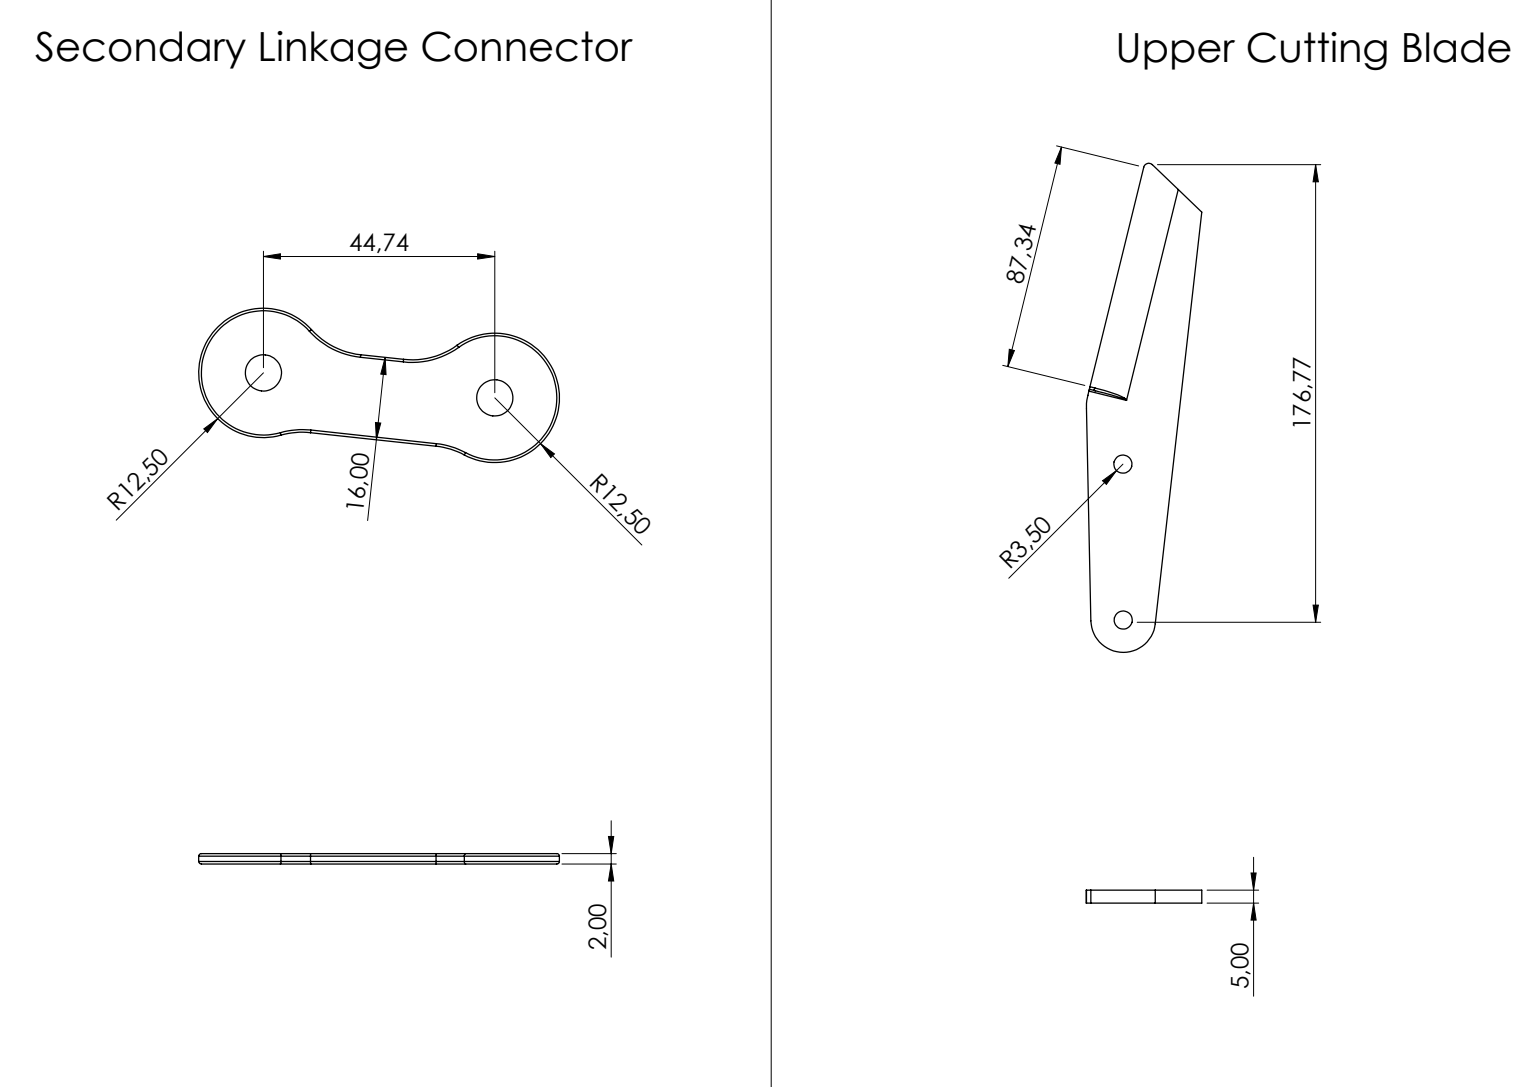
ISO-10303-21;
HEADER;
FILE_DESCRIPTION (('STEP AP214'),
    '1' );
FILE_NAME ('Secondary Linkage Connector.step',
    '2026-10-06T08:24:18',
    ( '' ),
    ( '' ),
    'SwSTEP 2.0',
    'SolidWorks 2020',
    '' );
FILE_SCHEMA (( 'AUTOMOTIVE_DESIGN' ));
ENDSEC;

DATA;
#3=AXIS2_PLACEMENT_3D ( 'NONE', #1835, #8382, #7525 ) ;
#18=CARTESIAN_POINT ( 'NONE',  ( -18.02719435607597021, -9.000000000000001776, -431.8467903975401896 ) ) ;
#24=VERTEX_POINT ( 'NONE', #8281 ) ;
#39=AXIS2_PLACEMENT_3D ( 'NONE', #1560, #10582, #8863 ) ;
#43=DIRECTION ( 'NONE',  ( 0.000000000000000000, -1.000000000000000000, 0.000000000000000000 ) ) ;
#51=CARTESIAN_POINT ( 'NONE',  ( -26.31853765676889267, -8.000000000000000000, -432.7407288192795249 ) ) ;
#69=CIRCLE ( 'NONE', #7777, 3.500000000000020428 ) ;
#75=ORIENTED_EDGE ( 'NONE', *, *, #5258, .T. ) ;
#94=EDGE_LOOP ( 'NONE', ( #5171, #2891 ) ) ;
#104=CARTESIAN_POINT ( 'NONE',  ( -46.74071243419621169, -8.000000000000000000, -414.3237589990241077 ) ) ;
#122=CARTESIAN_POINT ( 'NONE',  ( -46.74071243419621169, -8.000000000000000000, -414.3237589990241077 ) ) ;
#134=CYLINDRICAL_SURFACE ( 'NONE', #3984, 15.00000000000001776 ) ;
#162=ORIENTED_EDGE ( 'NONE', *, *, #3321, .F. ) ;
#168=VERTEX_POINT ( 'NONE', #2701 ) ;
#171=AXIS2_PLACEMENT_3D ( 'NONE', #4801, #2329, #8768 ) ;
#173=CYLINDRICAL_SURFACE ( 'NONE', #2650, 0.5000000000000004441 ) ;
#179=AXIS2_PLACEMENT_3D ( 'NONE', #8274, #10102, #4994 ) ;
#181=EDGE_CURVE ( 'NONE', #7240, #10131, #8649, .T. ) ;
#184=EDGE_CURVE ( 'NONE', #2293, #830, #6252, .T. ) ;
#204=CARTESIAN_POINT ( 'NONE',  ( -2.375181255485324439, -7.500000000000000888, -406.0201668106497550 ) ) ;
#222=DIRECTION ( 'NONE',  ( -0.9620620651437388204, 0.000000000000000000, 0.2728306852451987674 ) ) ;
#224=CARTESIAN_POINT ( 'NONE',  ( -48.08064548948741646, -8.000000000000000000, -401.8957833228595860 ) ) ;
#243=ORIENTED_EDGE ( 'NONE', *, *, #9605, .T. ) ;
#259=DIRECTION ( 'NONE',  ( -0.4716280258120416069, 0.000000000000000000, 0.8817975988108813779 ) ) ;
#262=AXIS2_PLACEMENT_3D ( 'NONE', #8998, #1740, #3461 ) ;
#280=DIRECTION ( 'NONE',  ( 0.000000000000000000, 1.000000000000000000, 0.000000000000000000 ) ) ;
#282=DIRECTION ( 'NONE',  ( 0.000000000000000000, 1.000000000000000000, 0.000000000000000000 ) ) ;
#295=PRODUCT_DEFINITION_SHAPE ( 'NONE', 'NONE',  #6660 ) ;
#318=ADVANCED_FACE ( 'NONE', ( #569 ), #2142, .T. ) ;
#322=ORIENTED_EDGE ( 'NONE', *, *, #2909, .F. ) ;
#329=ADVANCED_FACE ( 'NONE', ( #9439 ), #3687, .F. ) ;
#335=CIRCLE ( 'NONE', #1709, 15.00000000000001776 ) ;
#343=CARTESIAN_POINT ( 'NONE',  ( -43.33032886859687949, -9.000000000000001776, -402.2979831847329706 ) ) ;
#346=AXIS2_PLACEMENT_3D ( 'NONE', #860, #2744, #910 ) ;
#359=DIRECTION ( 'NONE',  ( 0.000000000000000000, 1.000000000000000000, 0.000000000000000000 ) ) ;
#372=CIRCLE ( 'NONE', #1744, 14.99999999999999467 ) ;
#384=LINE ( 'NONE', #2047, #7288 ) ;
#396=DIRECTION ( 'NONE',  ( -0.1071946444232961260, 0.000000000000000000, 0.9942380540931650135 ) ) ;
#398=ORIENTED_EDGE ( 'NONE', *, *, #3468, .T. ) ;
#410=FILL_AREA_STYLE_COLOUR ( '', #1992 ) ;
#421=STYLED_ITEM ( 'NONE', ( #698 ), #5138 ) ;
#451=CARTESIAN_POINT ( 'NONE',  ( -14.96977070983867009, -9.000000000000001776, -385.2505660326773409 ) ) ;
#460=ORIENTED_EDGE ( 'NONE', *, *, #1348, .F. ) ;
#463=DIRECTION ( 'NONE',  ( 0.000000000000000000, 1.000000000000000000, 0.000000000000000000 ) ) ;
#477=ADVANCED_FACE ( 'NONE', ( #9646 ), #582, .T. ) ;
#505=ADVANCED_FACE ( 'NONE', ( #3252 ), #1591, .F. ) ;
#511=VECTOR ( 'NONE', #4805, 1000.000000000000000 ) ;
#517=FACE_OUTER_BOUND ( 'NONE', #2695, .T. ) ;
#533=DIRECTION ( 'NONE',  ( 0.000000000000000000, -1.000000000000000000, 0.000000000000000000 ) ) ;
#543=EDGE_CURVE ( 'NONE', #1717, #2787, #7203, .T. ) ;
#554=EDGE_CURVE ( 'NONE', #2675, #1542, #4062, .T. ) ;
#565=ORIENTED_EDGE ( 'NONE', *, *, #5258, .F. ) ;
#569=FACE_OUTER_BOUND ( 'NONE', #2442, .T. ) ;
#570=CIRCLE ( 'NONE', #6572, 15.50000000000002487 ) ;
#582=TOROIDAL_SURFACE ( 'NONE', #1960, 12.00000000000000000, 0.5000000000000000000 ) ;
#597=EDGE_CURVE ( 'NONE', #10408, #168, #5818, .T. ) ;
#620=ORIENTED_EDGE ( 'NONE', *, *, #682, .T. ) ;
#622=ORIENTED_EDGE ( 'NONE', *, *, #10050, .T. ) ;
#641=EDGE_CURVE ( 'NONE', #5506, #9376, #3255, .T. ) ;
#647=ORIENTED_EDGE ( 'NONE', *, *, #4458, .T. ) ;
#652=CIRCLE ( 'NONE', #5110, 12.50000000000002309 ) ;
#661=VERTEX_POINT ( 'NONE', #3239 ) ;
#668=LINE ( 'NONE', #3943, #1019 ) ;
#671=ORIENTED_EDGE ( 'NONE', *, *, #1195, .T. ) ;
#682=EDGE_CURVE ( 'NONE', #9376, #10131, #2383, .T. ) ;
#685=ORIENTED_EDGE ( 'NONE', *, *, #8921, .F. ) ;
#692=AXIS2_PLACEMENT_3D ( 'NONE', #6618, #5963, #1017 ) ;
#697=FACE_OUTER_BOUND ( 'NONE', #8610, .T. ) ;
#698=PRESENTATION_STYLE_ASSIGNMENT (( #6324 ) ) ;
#739=EDGE_LOOP ( 'NONE', ( #961, #10607, #7941, #3569 ) ) ;
#764=ORIENTED_EDGE ( 'NONE', *, *, #7485, .F. ) ;
#767=AXIS2_PLACEMENT_3D ( 'NONE', #8861, #5631, #3922 ) ;
#775=AXIS2_PLACEMENT_3D ( 'NONE', #6193, #1570, #9735 ) ;
#780=EDGE_LOOP ( 'NONE', ( #4389, #3578, #5980, #685 ) ) ;
#784=STYLED_ITEM ( 'NONE', ( #5890 ), #966 ) ;
#801=DIRECTION ( 'NONE',  ( -0.9942380540931650135, 0.000000000000000000, -0.1071946444232960011 ) ) ;
#809=DIRECTION ( 'NONE',  ( 0.000000000000000000, 1.000000000000000000, 0.000000000000000000 ) ) ;
#814=DIRECTION ( 'NONE',  ( -0.4716280258120419955, 0.000000000000000000, 0.8817975988108811558 ) ) ;
#830=VERTEX_POINT ( 'NONE', #9310 ) ;
#832=DIRECTION ( 'NONE',  ( -0.5969176327498910695, 0.000000000000000000, -0.8023025238102309276 ) ) ;
#844=CARTESIAN_POINT ( 'NONE',  ( -27.92645732311833129, -8.000000000000000000, -417.8271580078820762 ) ) ;
#854=ORIENTED_EDGE ( 'NONE', *, *, #8756, .F. ) ;
#860=CARTESIAN_POINT ( 'NONE',  ( -37.82921798586427542, -8.000000000000000000, -422.3602549205905916 ) ) ;
#881=DIRECTION ( 'NONE',  ( 1.235123114895485641E-12, 1.000000000000000000, 4.329869796038106469E-12 ) ) ;
#882=DIRECTION ( 'NONE',  ( 0.000000000000000000, -1.000000000000000000, 0.000000000000000000 ) ) ;
#893=DIRECTION ( 'NONE',  ( 0.000000000000000000, 1.000000000000000000, 0.000000000000000000 ) ) ;
#899=EDGE_CURVE ( 'NONE', #830, #7069, #5948, .T. ) ;
#905=ORIENTED_EDGE ( 'NONE', *, *, #10218, .F. ) ;
#910=DIRECTION ( 'NONE',  ( 0.000000000000000000, 1.000000000000000000, 0.000000000000000000 ) ) ;
#911=VERTEX_POINT ( 'NONE', #2564 ) ;
#924=AXIS2_PLACEMENT_3D ( 'NONE', #8563, #5191, #9486 ) ;
#930=ORIENTED_EDGE ( 'NONE', *, *, #1348, .T. ) ;
#945=CARTESIAN_POINT ( 'NONE',  ( -2.000000000003786749, -9.500000000000001776, -409.4999999999758415 ) ) ;
#950=FACE_OUTER_BOUND ( 'NONE', #7230, .T. ) ;
#961=ORIENTED_EDGE ( 'NONE', *, *, #4838, .F. ) ;
#966=ADVANCED_BREP_SHAPE_REPRESENTATION ( '', ( #5138, #2817 ), #4734 ) ;
#1013=ADVANCED_FACE ( 'NONE', ( #6200 ), #2833, .T. ) ;
#1017=DIRECTION ( 'NONE',  ( 0.000000000000000000, 1.000000000000000000, 0.000000000000000000 ) ) ;
#1019=VECTOR ( 'NONE', #2386, 1000.000000000000000 ) ;
#1026=CARTESIAN_POINT ( 'NONE',  ( -9.285088343672491362, -8.000000000000000000, -419.6576319988688510 ) ) ;
#1033=VERTEX_POINT ( 'NONE', #10135 ) ;
#1038=CARTESIAN_POINT ( 'NONE',  ( -46.74071243419621169, -7.500000000000000888, -414.3237589990241077 ) ) ;
#1060=AXIS2_PLACEMENT_3D ( 'NONE', #4551, #2843, #6059 ) ;
#1077=CARTESIAN_POINT ( 'NONE',  ( -26.31853765676889267, -9.000000000000001776, -432.7407288192795249 ) ) ;
#1081=FACE_OUTER_BOUND ( 'NONE', #780, .T. ) ;
#1089=CARTESIAN_POINT ( 'NONE',  ( -2.000000000003786749, -9.500000000000001776, -409.4999999999758415 ) ) ;
#1096=EDGE_CURVE ( 'NONE', #4161, #1542, #7598, .T. ) ;
#1109=APPLICATION_CONTEXT ( 'automotive_design' ) ;
#1123=LINE ( 'NONE', #1174, #4934 ) ;
#1134=CARTESIAN_POINT ( 'NONE',  ( -27.98005464532998232, -9.000000000000001776, -417.3300389808354680 ) ) ;
#1146=EDGE_CURVE ( 'NONE', #2810, #4863, #5556, .T. ) ;
#1160=EDGE_CURVE ( 'NONE', #2578, #830, #10540, .T. ) ;
#1164=SHAPE_REPRESENTATION_RELATIONSHIP ( 'NONE' , 'NONE' ,  #1739, #966 ) ;
#1174=CARTESIAN_POINT ( 'NONE',  ( -48.08064548948741646, -9.500000000000001776, -401.8957833228595860 ) ) ;
#1183=VECTOR ( 'NONE', #6630, 1000.000000000000114 ) ;
#1195=EDGE_CURVE ( 'NONE', #661, #9639, #384, .T. ) ;
#1203=EDGE_CURVE ( 'NONE', #10408, #6648, #4023, .T. ) ;
#1243=AXIS2_PLACEMENT_3D ( 'NONE', #4932, #8161, #8048 ) ;
#1259=VERTEX_POINT ( 'NONE', #9314 ) ;
#1260=CARTESIAN_POINT ( 'NONE',  ( -13.30825372127758399, -7.500000000000000888, -400.6612558711213410 ) ) ;
#1265=CARTESIAN_POINT ( 'NONE',  ( -1.624818744522249503, -7.500000000000000888, -412.9798331893018712 ) ) ;
#1269=VECTOR ( 'NONE', #6090, 1000.000000000000114 ) ;
#1311=EDGE_LOOP ( 'NONE', ( #3567, #5407, #5270, #3199 ) ) ;
#1314=DIRECTION ( 'NONE',  ( 0.1071946444232958900, 0.000000000000000000, -0.9942380540931649024 ) ) ;
#1328=ADVANCED_FACE ( 'NONE', ( #5111 ), #6816, .T. ) ;
#1336=CYLINDRICAL_SURFACE ( 'NONE', #1965, 15.00000000000002309 ) ;
#1342=EDGE_LOOP ( 'NONE', ( #4527, #6060, #10354, #3368 ) ) ;
#1348=EDGE_CURVE ( 'NONE', #2010, #1489, #7829, .T. ) ;
#1356=AXIS2_PLACEMENT_3D ( 'NONE', #3266, #7300, #8854 ) ;
#1382=ORIENTED_EDGE ( 'NONE', *, *, #8963, .F. ) ;
#1392=AXIS2_PLACEMENT_3D ( 'NONE', #122, #8875, #3183 ) ;
#1403=CIRCLE ( 'NONE', #3292, 15.50000000000001421 ) ;
#1411=AXIS2_PLACEMENT_3D ( 'NONE', #1089, #7596, #5176 ) ;
#1426=EDGE_CURVE ( 'NONE', #10492, #1542, #5215, .T. ) ;
#1442=AXIS2_PLACEMENT_3D ( 'NONE', #2258, #3714, #7049 ) ;
#1449=AXIS2_PLACEMENT_3D ( 'NONE', #2696, #4307, #9306 ) ;
#1453=ORIENTED_EDGE ( 'NONE', *, *, #7309, .T. ) ;
#1462=DIRECTION ( 'NONE',  ( 0.000000000000000000, -1.000000000000000000, 0.000000000000000000 ) ) ;
#1486=CARTESIAN_POINT ( 'NONE',  ( -2.000000000003786749, -7.500000000000000888, -409.4999999999758415 ) ) ;
#1489=VERTEX_POINT ( 'NONE', #10527 ) ;
#1523=DIRECTION ( 'NONE',  ( 0.000000000000000000, 1.000000000000000000, 0.000000000000000000 ) ) ;
#1542=VERTEX_POINT ( 'NONE', #6029 ) ;
#1555=DIRECTION ( 'NONE',  ( 0.000000000000000000, 1.000000000000000000, 0.000000000000000000 ) ) ;
#1558=DIRECTION ( 'NONE',  ( 0.5828070674935411644, 0.000000000000000000, 0.8126105599114368250 ) ) ;
#1560=CARTESIAN_POINT ( 'NONE',  ( -2.000000000003786749, -7.500000000000000888, -409.4999999999758415 ) ) ;
#1570=DIRECTION ( 'NONE',  ( 0.000000000000000000, 1.000000000000000000, 0.000000000000000000 ) ) ;
#1581=CIRCLE ( 'NONE', #2784, 0.5000000000000004441 ) ;
#1591=CYLINDRICAL_SURFACE ( 'NONE', #6329, 3.500000000000020428 ) ;
#1611=FACE_BOUND ( 'NONE', #3102, .T. ) ;
#1613=( NAMED_UNIT ( * ) PLANE_ANGLE_UNIT ( ) SI_UNIT ( $, .RADIAN. ) );
#1624=CARTESIAN_POINT ( 'NONE',  ( -14.96977070983867009, -9.000000000000001776, -385.2505660326773409 ) ) ;
#1652=DIRECTION ( 'NONE',  ( -0.1071946444232959594, 0.000000000000000000, 0.9942380540931649024 ) ) ;
#1655=EDGE_LOOP ( 'NONE', ( #322, #8238, #1851, #243 ) ) ;
#1662=FACE_BOUND ( 'NONE', #3043, .T. ) ;
#1678=AXIS2_PLACEMENT_3D ( 'NONE', #9635, #3832, #396 ) ;
#1690=DIRECTION ( 'NONE',  ( 0.1071946444232947937, 0.000000000000000000, -0.9942380540931651245 ) ) ;
#1694=EDGE_CURVE ( 'NONE', #7772, #4372, #1906, .T. ) ;
#1709=AXIS2_PLACEMENT_3D ( 'NONE', #18, #1523, #3137 ) ;
#1710=VECTOR ( 'NONE', #4006, 1000.000000000000000 ) ;
#1717=VERTEX_POINT ( 'NONE', #3883 ) ;
#1739=SHAPE_REPRESENTATION ( 'Secondary Linkage Connector', ( #2817 ), #4734 ) ;
#1740=DIRECTION ( 'NONE',  ( 0.000000000000000000, 1.000000000000000000, 0.000000000000000000 ) ) ;
#1744=AXIS2_PLACEMENT_3D ( 'NONE', #451, #8713, #4585 ) ;
#1770=ORIENTED_EDGE ( 'NONE', *, *, #4366, .T. ) ;
#1782=AXIS2_PLACEMENT_3D ( 'NONE', #9436, #9485, #2981 ) ;
#1788=TOROIDAL_SURFACE ( 'NONE', #9510, 15.50000000000000000, 0.5000000000000000000 ) ;
#1795=AXIS2_PLACEMENT_3D ( 'NONE', #9777, #7308, #1558 ) ;
#1825=LINE ( 'NONE', #5841, #9195 ) ;
#1835=CARTESIAN_POINT ( 'NONE',  ( -37.82921798586427542, -9.000000000000001776, -422.3602549205905916 ) ) ;
#1851=ORIENTED_EDGE ( 'NONE', *, *, #10227, .T. ) ;
#1858=AXIS2_PLACEMENT_3D ( 'NONE', #7847, #8650, #4626 ) ;
#1861=ORIENTED_EDGE ( 'NONE', *, *, #7909, .T. ) ;
#1880=EDGE_CURVE ( 'NONE', #10437, #4923, #3628, .T. ) ;
#1888=VECTOR ( 'NONE', #9928, 1000.000000000000000 ) ;
#1904=DIRECTION ( 'NONE',  ( -0.5828070674935416084, 0.000000000000000000, -0.8126105599114364919 ) ) ;
#1906=CIRCLE ( 'NONE', #4643, 0.5000000000000004441 ) ;
#1921=ADVANCED_FACE ( 'NONE', ( #4094 ), #2768, .T. ) ;
#1942=DIRECTION ( 'NONE',  ( -0.8126105599114364919, 6.772514207610136972E-17, 0.5828070674935419415 ) ) ;
#1945=AXIS2_PLACEMENT_3D ( 'NONE', #7118, #3996, #10385 ) ;
#1960=AXIS2_PLACEMENT_3D ( 'NONE', #9757, #2288, #832 ) ;
#1965=AXIS2_PLACEMENT_3D ( 'NONE', #2797, #6170, #4507 ) ;
#1971=ORIENTED_EDGE ( 'NONE', *, *, #10530, .T. ) ;
#1975=CIRCLE ( 'NONE', #4723, 15.50000000000001421 ) ;
#1978=SURFACE_SIDE_STYLE ('',( #6922 ) ) ;
#1989=CARTESIAN_POINT ( 'NONE',  ( -1.624818744522249503, -7.500000000000000888, -412.9798331893018712 ) ) ;
#1990=CARTESIAN_POINT ( 'NONE',  ( -47.11589368967775471, -7.500000000000000888, -410.8439258096980780 ) ) ;
#1992=COLOUR_RGB ( '', 0.31764706, 0.68627451, 0.89019608) ;
#2010=VERTEX_POINT ( 'NONE', #4526 ) ;
#2013=EDGE_CURVE ( 'NONE', #9376, #2675, #372, .T. ) ;
#2022=CARTESIAN_POINT ( 'NONE',  ( -46.74071243419621169, -9.500000000000001776, -414.3237589990241077 ) ) ;
#2037=ADVANCED_FACE ( 'NONE', ( #2063 ), #7167, .T. ) ;
#2042=FACE_OUTER_BOUND ( 'NONE', #7532, .T. ) ;
#2047=CARTESIAN_POINT ( 'NONE',  ( -13.30825372127758399, -9.500000000000001776, -400.6612558711213410 ) ) ;
#2050=AXIS2_PLACEMENT_3D ( 'NONE', #9959, #2545, #7644 ) ;
#2058=ORIENTED_EDGE ( 'NONE', *, *, #6274, .F. ) ;
#2059=CARTESIAN_POINT ( 'NONE',  ( -37.62994892358009480, -8.000000000000000000, -402.7806230189665371 ) ) ;
#2063=FACE_OUTER_BOUND ( 'NONE', #3743, .T. ) ;
#2101=EDGE_LOOP ( 'NONE', ( #7660, #1453, #460, #3857 ) ) ;
#2121=CIRCLE ( 'NONE', #9340, 12.49999999999998934 ) ;
#2122=EDGE_LOOP ( 'NONE', ( #565, #7254, #9589, #2187 ) ) ;
#2123=CARTESIAN_POINT ( 'NONE',  ( -19.63511402242740189, -9.000000000000001776, -416.9332195861429113 ) ) ;
#2136=ORIENTED_EDGE ( 'NONE', *, *, #597, .T. ) ;
#2141=CIRCLE ( 'NONE', #1449, 12.49999999999998934 ) ;
#2142=TOROIDAL_SURFACE ( 'NONE', #4724, 15.50000000000000000, 0.5000000000000000000 ) ;
#2144=DIRECTION ( 'NONE',  ( 0.000000000000000000, 1.000000000000000000, 0.000000000000000000 ) ) ;
#2169=DIRECTION ( 'NONE',  ( 0.000000000000000000, 1.000000000000000000, 0.000000000000000000 ) ) ;
#2187=ORIENTED_EDGE ( 'NONE', *, *, #1880, .F. ) ;
#2199=CARTESIAN_POINT ( 'NONE',  ( -19.53582934753526246, -8.000000000000000000, -416.4196174530124495 ) ) ;
#2202=ADVANCED_FACE ( 'NONE', ( #8340 ), #10258, .T. ) ;
#2226=CIRCLE ( 'NONE', #2050, 0.5000000000000004441 ) ;
#2229=ORIENTED_EDGE ( 'NONE', *, *, #7954, .F. ) ;
#2244=AXIS2_PLACEMENT_3D ( 'NONE', #6985, #4554, #7828 ) ;
#2258=CARTESIAN_POINT ( 'NONE',  ( -13.30825372127758399, -8.000000000000000000, -400.6612558711213410 ) ) ;
#2280=DIRECTION ( 'NONE',  ( -0.1071946444232947937, 0.000000000000000000, 0.9942380540931651245 ) ) ;
#2288=DIRECTION ( 'NONE',  ( 0.000000000000000000, 1.000000000000000000, 0.000000000000000000 ) ) ;
#2293=VERTEX_POINT ( 'NONE', #8541 ) ;
#2296=ORIENTED_EDGE ( 'NONE', *, *, #6736, .F. ) ;
#2303=DIRECTION ( 'NONE',  ( 0.7508065140037780694, 0.000000000000000000, -0.6605222013903048195 ) ) ;
#2307=DIRECTION ( 'NONE',  ( 0.000000000000000000, -1.000000000000000000, 0.000000000000000000 ) ) ;
#2309=VECTOR ( 'NONE', #9307, 1000.000000000000114 ) ;
#2310=EDGE_LOOP ( 'NONE', ( #7345, #2928, #3923, #8777 ) ) ;
#2312=CIRCLE ( 'NONE', #8147, 15.00000000000001776 ) ;
#2327=ORIENTED_EDGE ( 'NONE', *, *, #5504, .F. ) ;
#2329=DIRECTION ( 'NONE',  ( 0.000000000000000000, -1.000000000000000000, 0.000000000000000000 ) ) ;
#2344=DIRECTION ( 'NONE',  ( 0.000000000000000000, -1.000000000000000000, 0.000000000000000000 ) ) ;
#2346=EDGE_CURVE ( 'NONE', #5580, #3896, #652, .T. ) ;
#2361=DIRECTION ( 'NONE',  ( 0.000000000000000000, 1.000000000000000000, 0.000000000000000000 ) ) ;
#2374=PRODUCT_CONTEXT ( 'NONE', #6331, 'mechanical' ) ;
#2376=DIRECTION ( 'NONE',  ( -1.908117741397742798E-11, 1.000000000000000000, -2.057253813257758150E-12 ) ) ;
#2383=LINE ( 'NONE', #7908, #3600 ) ;
#2386=DIRECTION ( 'NONE',  ( 0.000000000000000000, 1.000000000000000000, 0.000000000000000000 ) ) ;
#2401=EDGE_LOOP ( 'NONE', ( #2136, #9614, #2229, #5792 ) ) ;
#2404=ORIENTED_EDGE ( 'NONE', *, *, #1426, .T. ) ;
#2415=PLANE ( 'NONE',  #9955 ) ;
#2436=ORIENTED_EDGE ( 'NONE', *, *, #7339, .F. ) ;
#2439=VECTOR ( 'NONE', #3583, 1000.000000000000000 ) ;
#2442=EDGE_LOOP ( 'NONE', ( #8291, #3143, #9082, #10187 ) ) ;
#2451=EDGE_CURVE ( 'NONE', #24, #10408, #6657, .T. ) ;
#2466=CARTESIAN_POINT ( 'NONE',  ( -43.33032886859687949, -9.000000000000001776, -402.2979831847329706 ) ) ;
#2470=FACE_OUTER_BOUND ( 'NONE', #8150, .T. ) ;
#2481=CLOSED_SHELL ( 'NONE', ( #6399, #2037, #5406, #10272, #3571, #4819, #505, #7275, #10422, #2202, #8950, #8172, #9099, #1013, #6359, #4140, #329, #1921, #3048, #6808, #3575, #4250, #9302, #9900, #9238, #477, #8750, #10156, #1328, #7265, #318, #5097, #8841, #8169 ) ) ;
#2482=CARTESIAN_POINT ( 'NONE',  ( -19.68871134463705985, -7.500000000000000888, -416.4361005590961327 ) ) ;
#2486=EDGE_LOOP ( 'NONE', ( #8430, #75, #5442, #5537 ) ) ;
#2489=CIRCLE ( 'NONE', #3689, 12.50000000000001421 ) ;
#2501=ORIENTED_EDGE ( 'NONE', *, *, #3654, .F. ) ;
#2544=AXIS2_PLACEMENT_3D ( 'NONE', #6737, #6079, #4316 ) ;
#2545=DIRECTION ( 'NONE',  ( -0.9942380540931650135, 0.000000000000000000, -0.1071946444232960011 ) ) ;
#2563=DIRECTION ( 'NONE',  ( 0.000000000000000000, -1.000000000000000000, 0.000000000000000000 ) ) ;
#2564=CARTESIAN_POINT ( 'NONE',  ( -37.82921798586438911, -9.500000000000001776, -422.3602549205895684 ) ) ;
#2578=VERTEX_POINT ( 'NONE', #9303 ) ;
#2580=VECTOR ( 'NONE', #5428, 1000.000000000000000 ) ;
#2587=ORIENTED_EDGE ( 'NONE', *, *, #3654, .T. ) ;
#2606=FACE_OUTER_BOUND ( 'NONE', #2310, .T. ) ;
#2626=SURFACE_STYLE_USAGE ( .BOTH. , #1978 ) ;
#2641=ORIENTED_EDGE ( 'NONE', *, *, #10218, .T. ) ;
#2648=ORIENTED_EDGE ( 'NONE', *, *, #899, .T. ) ;
#2650=AXIS2_PLACEMENT_3D ( 'NONE', #2199, #3708, #8535 ) ;
#2662=MECHANICAL_DESIGN_GEOMETRIC_PRESENTATION_REPRESENTATION('',(#421),#4379);
#2675=VERTEX_POINT ( 'NONE', #9253 ) ;
#2683=EDGE_CURVE ( 'NONE', #5580, #4923, #1123, .T. ) ;
#2695=EDGE_LOOP ( 'NONE', ( #10232, #9170, #8030, #5805 ) ) ;
#2696=CARTESIAN_POINT ( 'NONE',  ( -2.000000000003786749, -8.000000000000000000, -409.4999999999758415 ) ) ;
#2697=AXIS2_PLACEMENT_3D ( 'NONE', #6841, #10009, #5264 ) ;
#2699=CARTESIAN_POINT ( 'NONE',  ( -3.339933055294988851, -9.000000000000001776, -397.0720243238112630 ) ) ;
#2701=CARTESIAN_POINT ( 'NONE',  ( -43.33032886862778099, -8.000000000000000000, -402.2979831847262631 ) ) ;
#2724=ORIENTED_EDGE ( 'NONE', *, *, #3777, .T. ) ;
#2726=DIRECTION ( 'NONE',  ( -0.1071946444232964035, 0.000000000000000000, 0.9942380540931649024 ) ) ;
#2740=CIRCLE ( 'NONE', #1356, 12.49999999999998934 ) ;
#2744=DIRECTION ( 'NONE',  ( -0.6697079934638360266, 0.000000000000000000, -0.7426245373610022016 ) ) ;
#2747=CARTESIAN_POINT ( 'NONE',  ( -37.57635160138833896, -7.500000000000000888, -403.2777420460153053 ) ) ;
#2768=TOROIDAL_SURFACE ( 'NONE', #8769, 15.50000000000000000, 0.5000000000000000000 ) ;
#2775=DIRECTION ( 'NONE',  ( 0.000000000000000000, -1.000000000000000000, 0.000000000000000000 ) ) ;
#2784=AXIS2_PLACEMENT_3D ( 'NONE', #8277, #1942, #4205 ) ;
#2787=VERTEX_POINT ( 'NONE', #8633 ) ;
#2789=ORIENTED_EDGE ( 'NONE', *, *, #899, .F. ) ;
#2794=DIRECTION ( 'NONE',  ( 0.2728306852451984343, 0.000000000000000000, 0.9620620651437388204 ) ) ;
#2797=CARTESIAN_POINT ( 'NONE',  ( -26.31853765676889267, -9.633703999999999823, -432.7407288192795249 ) ) ;
#2810=VERTEX_POINT ( 'NONE', #1989 ) ;
#2817=AXIS2_PLACEMENT_3D ( 'NONE', #8634, #3966, #3161 ) ;
#2823=CIRCLE ( 'NONE', #8826, 15.00000000000001776 ) ;
#2833=CYLINDRICAL_SURFACE ( 'NONE', #924, 12.49999999999998757 ) ;
#2842=ORIENTED_EDGE ( 'NONE', *, *, #5598, .F. ) ;
#2843=DIRECTION ( 'NONE',  ( 0.000000000000000000, 1.000000000000000000, 0.000000000000000000 ) ) ;
#2852=DIRECTION ( 'NONE',  ( 0.000000000000000000, -1.000000000000000000, 0.000000000000000000 ) ) ;
#2866=ORIENTED_EDGE ( 'NONE', *, *, #7339, .T. ) ;
#2881=DIRECTION ( 'NONE',  ( 0.1173809667161562209, 0.000000000000000000, -0.9930869592602555862 ) ) ;
#2891=ORIENTED_EDGE ( 'NONE', *, *, #543, .F. ) ;
#2893=CARTESIAN_POINT ( 'NONE',  ( -39.23786858994942151, -8.000000000000000000, -387.8670522075712483 ) ) ;
#2909=EDGE_CURVE ( 'NONE', #2810, #1259, #8675, .T. ) ;
#2910=DIRECTION ( 'NONE',  ( 0.1071946444232954182, 0.000000000000000000, -0.9942380540931651245 ) ) ;
#2923=AXIS2_PLACEMENT_3D ( 'NONE', #2893, #9207, #8737 ) ;
#2928=ORIENTED_EDGE ( 'NONE', *, *, #10338, .F. ) ;
#2981=DIRECTION ( 'NONE',  ( -0.1071946444232958900, 0.000000000000000000, 0.9942380540931649024 ) ) ;
#3026=CARTESIAN_POINT ( 'NONE',  ( -37.62994892359998289, -8.000000000000000000, -402.7806230189686971 ) ) ;
#3043=EDGE_LOOP ( 'NONE', ( #7539, #5201 ) ) ;
#3048=ADVANCED_FACE ( 'NONE', ( #1081 ), #6843, .T. ) ;
#3051=LINE ( 'NONE', #6219, #4361 ) ;
#3053=CARTESIAN_POINT ( 'NONE',  ( -46.74071243419621169, -8.000000000000000000, -414.3237589990241077 ) ) ;
#3056=SURFACE_SIDE_STYLE ('',( #10414 ) ) ;
#3073=ORIENTED_EDGE ( 'NONE', *, *, #597, .F. ) ;
#3077=VERTEX_POINT ( 'NONE', #8542 ) ;
#3081=CIRCLE ( 'NONE', #7887, 0.5000000000000004441 ) ;
#3102=EDGE_LOOP ( 'NONE', ( #6612, #162 ) ) ;
#3110=ORIENTED_EDGE ( 'NONE', *, *, #7485, .T. ) ;
#3125=EDGE_CURVE ( 'NONE', #6593, #7069, #10600, .T. ) ;
#3137=DIRECTION ( 'NONE',  ( -0.1071946444232958900, 0.000000000000000000, 0.9942380540931649024 ) ) ;
#3143=ORIENTED_EDGE ( 'NONE', *, *, #10338, .T. ) ;
#3152=ORIENTED_EDGE ( 'NONE', *, *, #682, .F. ) ;
#3154=CARTESIAN_POINT ( 'NONE',  ( -7.895350322666780940, -9.000000000000001776, -398.4775300148504016 ) ) ;
#3161=DIRECTION ( 'NONE',  ( 1.000000000000000000, 0.000000000000000000, 0.000000000000000000 ) ) ;
#3169=ORIENTED_EDGE ( 'NONE', *, *, #3440, .F. ) ;
#3183=DIRECTION ( 'NONE',  ( 0.7426245373610016465, 0.000000000000000000, -0.6697079934638365817 ) ) ;
#3194=VERTEX_POINT ( 'NONE', #8590 ) ;
#3199=ORIENTED_EDGE ( 'NONE', *, *, #6021, .F. ) ;
#3219=DIRECTION ( 'NONE',  ( 0.1071946444232959872, 0.000000000000000000, -0.9942380540931649024 ) ) ;
#3232=FACE_OUTER_BOUND ( 'NONE', #2101, .T. ) ;
#3239=CARTESIAN_POINT ( 'NONE',  ( -13.30825372127758399, -9.500000000000001776, -400.6612558711213410 ) ) ;
#3252=FACE_OUTER_BOUND ( 'NONE', #1655, .T. ) ;
#3253=CARTESIAN_POINT ( 'NONE',  ( -19.63511402242541237, -8.000000000000000000, -416.9332195861426840 ) ) ;
#3255=CIRCLE ( 'NONE', #171, 12.50000000000001421 ) ;
#3266=CARTESIAN_POINT ( 'NONE',  ( -2.000000000003786749, -8.000000000000000000, -409.4999999999758415 ) ) ;
#3290=ORIENTED_EDGE ( 'NONE', *, *, #5385, .T. ) ;
#3292=AXIS2_PLACEMENT_3D ( 'NONE', #9308, #9094, #4410 ) ;
#3312=DIRECTION ( 'NONE',  ( 0.000000000000000000, -1.000000000000000000, 0.000000000000000000 ) ) ;
#3313=AXIS2_PLACEMENT_3D ( 'NONE', #4697, #9693, #2280 ) ;
#3321=EDGE_CURVE ( 'NONE', #1259, #3194, #7259, .T. ) ;
#3327=ORIENTED_EDGE ( 'NONE', *, *, #8756, .T. ) ;
#3343=CARTESIAN_POINT ( 'NONE',  ( -46.74071243419621169, -9.500000000000001776, -414.3237589990241077 ) ) ;
#3368=ORIENTED_EDGE ( 'NONE', *, *, #10050, .F. ) ;
#3381=DIRECTION ( 'NONE',  ( 0.000000000000000000, -1.000000000000000000, 0.000000000000000000 ) ) ;
#3407=ORIENTED_EDGE ( 'NONE', *, *, #9625, .F. ) ;
#3417=CARTESIAN_POINT ( 'NONE',  ( -8.993684809926110191, -7.500000000000000888, -419.2513267189134467 ) ) ;
#3420=ORIENTED_EDGE ( 'NONE', *, *, #1146, .F. ) ;
#3426=AXIS2_PLACEMENT_3D ( 'NONE', #9072, #43, #9879 ) ;
#3431=CARTESIAN_POINT ( 'NONE',  ( -14.96977070983867009, -8.000000000000000000, -385.2505660326773409 ) ) ;
#3438=ORIENTED_EDGE ( 'NONE', *, *, #6940, .F. ) ;
#3440=EDGE_CURVE ( 'NONE', #6553, #5580, #10334, .T. ) ;
#3461=DIRECTION ( 'NONE',  ( -0.4824394482813016416, 0.000000000000000000, 0.8759293229148304993 ) ) ;
#3468=EDGE_CURVE ( 'NONE', #5957, #2787, #9355, .T. ) ;
#3483=CIRCLE ( 'NONE', #6565, 12.50000000000001421 ) ;
#3488=TOROIDAL_SURFACE ( 'NONE', #9326, 15.50000000000000000, 0.5000000000000000000 ) ;
#3508=CARTESIAN_POINT ( 'NONE',  ( -8.993684809926110191, -9.000000000000001776, -419.2513267189134467 ) ) ;
#3512=CARTESIAN_POINT ( 'NONE',  ( -46.74071243419621169, -9.000000000000001776, -414.3237589990241077 ) ) ;
#3517=ORIENTED_EDGE ( 'NONE', *, *, #6082, .F. ) ;
#3532=ORIENTED_EDGE ( 'NONE', *, *, #8111, .T. ) ;
#3534=DIRECTION ( 'NONE',  ( 0.000000000000000000, 1.000000000000000000, 0.000000000000000000 ) ) ;
#3536=EDGE_CURVE ( 'NONE', #6553, #168, #9721, .T. ) ;
#3541=DIRECTION ( 'NONE',  ( 0.7426245373610016465, 0.000000000000000000, -0.6697079934638365817 ) ) ;
#3564=AXIS2_PLACEMENT_3D ( 'NONE', #8918, #5528, #5635 ) ;
#3567=ORIENTED_EDGE ( 'NONE', *, *, #7921, .T. ) ;
#3569=ORIENTED_EDGE ( 'NONE', *, *, #1096, .F. ) ;
#3571=ADVANCED_FACE ( 'NONE', ( #4883 ), #6381, .F. ) ;
#3575=ADVANCED_FACE ( 'NONE', ( #8209 ), #8789, .T. ) ;
#3578=ORIENTED_EDGE ( 'NONE', *, *, #1096, .T. ) ;
#3583=DIRECTION ( 'NONE',  ( 9.254477013072932692E-13, 1.000000000000000000, 9.977795243863814969E-14 ) ) ;
#3599=TOROIDAL_SURFACE ( 'NONE', #6328, 12.00000000000000000, 0.5000000000000000000 ) ;
#3600=VECTOR ( 'NONE', #5647, 1000.000000000000000 ) ;
#3622=CARTESIAN_POINT ( 'NONE',  ( -2.000000000003786749, -9.500000000000001776, -409.4999999999758415 ) ) ;
#3628=CIRCLE ( 'NONE', #1392, 12.50000000000001243 ) ;
#3654=EDGE_CURVE ( 'NONE', #1489, #3077, #3483, .T. ) ;
#3666=ORIENTED_EDGE ( 'NONE', *, *, #5598, .T. ) ;
#3675=AXIS2_PLACEMENT_3D ( 'NONE', #1134, #7690, #10109 ) ;
#3677=CIRCLE ( 'NONE', #1795, 15.00000000000002487 ) ;
#3683=LINE ( 'NONE', #2123, #2439 ) ;
#3687=CYLINDRICAL_SURFACE ( 'NONE', #4890, 14.99999999999999467 ) ;
#3689=AXIS2_PLACEMENT_3D ( 'NONE', #9599, #3959, #7239 ) ;
#3703=FACE_BOUND ( 'NONE', #94, .T. ) ;
#3708=DIRECTION ( 'NONE',  ( -0.9942380540931650135, 0.000000000000000000, -0.1071946444232960011 ) ) ;
#3713=CARTESIAN_POINT ( 'NONE',  ( -7.659536309752155603, -8.000000000000000000, -398.9184288142485570 ) ) ;
#3714=DIRECTION ( 'NONE',  ( 0.9942380540931650135, 0.000000000000000000, 0.1071946444232960011 ) ) ;
#3723=ORIENTED_EDGE ( 'NONE', *, *, #3440, .T. ) ;
#3732=ORIENTED_EDGE ( 'NONE', *, *, #1203, .T. ) ;
#3741=CARTESIAN_POINT ( 'NONE',  ( -45.40077937890500692, -9.500000000000001776, -426.7517346751886862 ) ) ;
#3743=EDGE_LOOP ( 'NONE', ( #3841, #3110, #8398, #3152 ) ) ;
#3751=CARTESIAN_POINT ( 'NONE',  ( -46.74071243419621169, -9.500000000000001776, -414.3237589990241077 ) ) ;
#3761=AXIS2_PLACEMENT_3D ( 'NONE', #9004, #6690, #881 ) ;
#3766=LINE ( 'NONE', #5483, #7208 ) ;
#3777=EDGE_CURVE ( 'NONE', #4923, #168, #8279, .T. ) ;
#3779=CIRCLE ( 'NONE', #2244, 0.5000000000000004441 ) ;
#3832=DIRECTION ( 'NONE',  ( 0.000000000000000000, 1.000000000000000000, 0.000000000000000000 ) ) ;
#3841=ORIENTED_EDGE ( 'NONE', *, *, #641, .F. ) ;
#3857=ORIENTED_EDGE ( 'NONE', *, *, #5482, .F. ) ;
#3861=TOROIDAL_SURFACE ( 'NONE', #262, 12.00000000000000000, 0.5000000000000000000 ) ;
#3880=FACE_OUTER_BOUND ( 'NONE', #4914, .T. ) ;
#3883=CARTESIAN_POINT ( 'NONE',  ( -46.36553117871467578, -9.500000000000001776, -417.8035921883502510 ) ) ;
#3896=VERTEX_POINT ( 'NONE', #6923 ) ;
#3922=DIRECTION ( 'NONE',  ( -0.1071946444232959872, 0.000000000000000000, 0.9942380540931649024 ) ) ;
#3923=ORIENTED_EDGE ( 'NONE', *, *, #4838, .T. ) ;
#3932=CARTESIAN_POINT ( 'NONE',  ( -37.62994892356022092, -9.000000000000001776, -402.7806230189644339 ) ) ;
#3933=DIRECTION ( 'NONE',  ( -0.9942380540931649024, 0.000000000000000000, -0.1071946444232959872 ) ) ;
#3943=CARTESIAN_POINT ( 'NONE',  ( -0.6600669447125852018, -9.500000000000001776, -421.9279756761403632 ) ) ;
#3946=CIRCLE ( 'NONE', #7551, 11.99999999999998401 ) ;
#3959=DIRECTION ( 'NONE',  ( 0.000000000000000000, -1.000000000000000000, 0.000000000000000000 ) ) ;
#3966=DIRECTION ( 'NONE',  ( 0.000000000000000000, 0.000000000000000000, 1.000000000000000000 ) ) ;
#3984=AXIS2_PLACEMENT_3D ( 'NONE', #6746, #9965, #5867 ) ;
#3993=AXIS2_PLACEMENT_3D ( 'NONE', #6988, #6165, #2794 ) ;
#3996=DIRECTION ( 'NONE',  ( -0.1071946444232959872, 0.000000000000000000, 0.9942380540931649024 ) ) ;
#4006=DIRECTION ( 'NONE',  ( -4.096342363382135256E-11, 1.000000000000000000, -4.416507306988328157E-12 ) ) ;
#4015=ORIENTED_EDGE ( 'NONE', *, *, #3777, .F. ) ;
#4023=CIRCLE ( 'NONE', #2697, 15.49999999999999467 ) ;
#4025=CARTESIAN_POINT ( 'NONE',  ( -24.37035621709999944, -9.500000000000001776, -411.9118794995000030 ) ) ;
#4029=ORIENTED_EDGE ( 'NONE', *, *, #8616, .T. ) ;
#4032=ORIENTED_EDGE ( 'NONE', *, *, #2909, .T. ) ;
#4062=LINE ( 'NONE', #4816, #1710 ) ;
#4091=CARTESIAN_POINT ( 'NONE',  ( -46.74071243419621169, -7.500000000000000888, -414.3237589990241077 ) ) ;
#4092=DIRECTION ( 'NONE',  ( 0.4806425702415767498, 0.000000000000000000, -0.8769165978994644117 ) ) ;
#4094=FACE_OUTER_BOUND ( 'NONE', #7595, .T. ) ;
#4102=UNCERTAINTY_MEASURE_WITH_UNIT (LENGTH_MEASURE( 1.000000000000000082E-05 ), #6052, 'distance_accuracy_value', 'NONE');
#4111=AXIS2_PLACEMENT_3D ( 'NONE', #8207, #8043, #5729 ) ;
#4140=ADVANCED_FACE ( 'NONE', ( #8135 ), #5544, .T. ) ;
#4161=VERTEX_POINT ( 'NONE', #3026 ) ;
#4162=DIRECTION ( 'NONE',  ( 0.000000000000000000, -1.000000000000000000, 0.000000000000000000 ) ) ;
#4174=EDGE_CURVE ( 'NONE', #5957, #5389, #7940, .T. ) ;
#4175=DIRECTION ( 'NONE',  ( 0.000000000000000000, -1.000000000000000000, 0.000000000000000000 ) ) ;
#4179=CARTESIAN_POINT ( 'NONE',  ( -28.19723202891387359, -9.000000000000001776, -417.3534541501846888 ) ) ;
#4181=CYLINDRICAL_SURFACE ( 'NONE', #3426, 3.500000000000020428 ) ;
#4195=AXIS2_PLACEMENT_3D ( 'NONE', #8562, #6046, #1314 ) ;
#4205=DIRECTION ( 'NONE',  ( -1.318389841742372130E-13, 1.000000000000000000, -2.220446049250311061E-13 ) ) ;
#4229=CARTESIAN_POINT ( 'NONE',  ( -14.96977070983867009, -7.500000000000000888, -385.2505660326773409 ) ) ;
#4250=ADVANCED_FACE ( 'NONE', ( #8211 ), #3488, .T. ) ;
#4307=DIRECTION ( 'NONE',  ( 0.000000000000000000, 1.000000000000000000, 0.000000000000000000 ) ) ;
#4316=DIRECTION ( 'NONE',  ( 0.000000000000000000, 1.000000000000000000, 0.000000000000000000 ) ) ;
#4325=CARTESIAN_POINT ( 'NONE',  ( -27.98005464532998232, -7.500000000000000888, -417.3300389808354680 ) ) ;
#4327=DIRECTION ( 'NONE',  ( 0.1071946444232954182, 0.000000000000000000, -0.9942380540931651245 ) ) ;
#4336=AXIS2_PLACEMENT_3D ( 'NONE', #3622, #6030, #1904 ) ;
#4350=VERTEX_POINT ( 'NONE', #5198 ) ;
#4361=VECTOR ( 'NONE', #7943, 1000.000000000000000 ) ;
#4366=EDGE_CURVE ( 'NONE', #8504, #4350, #570, .T. ) ;
#4367=CIRCLE ( 'NONE', #10365, 12.50000000000001243 ) ;
#4372=VERTEX_POINT ( 'NONE', #8263 ) ;
#4378=AXIS2_PLACEMENT_3D ( 'NONE', #945, #3312, #5775 ) ;
#4379=( GEOMETRIC_REPRESENTATION_CONTEXT ( 3 ) GLOBAL_UNCERTAINTY_ASSIGNED_CONTEXT ( ( #5921 ) ) GLOBAL_UNIT_ASSIGNED_CONTEXT ( ( #9665, #1613, #6498 ) ) REPRESENTATION_CONTEXT ( 'NONE', 'WORKASPACE' ) );
#4389=ORIENTED_EDGE ( 'NONE', *, *, #7954, .T. ) ;
#4392=DIRECTION ( 'NONE',  ( -0.1071946444232947937, 0.000000000000000000, 0.9942380540931651245 ) ) ;
#4405=PRODUCT_DEFINITION_FORMATION_WITH_SPECIFIED_SOURCE ( 'ANY', '', #10331, .NOT_KNOWN. ) ;
#4410=DIRECTION ( 'NONE',  ( -0.1071946444232959594, 0.000000000000000000, 0.9942380540931649024 ) ) ;
#4417=PRODUCT_DEFINITION_CONTEXT ( 'detailed design', #1109, 'design' ) ;
#4419=ORIENTED_EDGE ( 'NONE', *, *, #181, .T. ) ;
#4439=CARTESIAN_POINT ( 'NONE',  ( -45.40077937890500692, -8.000000000000000000, -426.7517346751886862 ) ) ;
#4452=AXIS2_PLACEMENT_3D ( 'NONE', #9704, #2344, #5613 ) ;
#4455=DIRECTION ( 'NONE',  ( 0.2728306852451988784, 0.000000000000000000, 0.9620620651437385984 ) ) ;
#4458=EDGE_CURVE ( 'NONE', #1542, #10131, #2823, .T. ) ;
#4489=EDGE_CURVE ( 'NONE', #7069, #6915, #2312, .T. ) ;
#4507=DIRECTION ( 'NONE',  ( -0.7426245373610013134, 0.000000000000000000, 0.6697079934638370258 ) ) ;
#4510=DIRECTION ( 'NONE',  ( 0.8817975988108817109, 0.000000000000000000, 0.4716280258120411073 ) ) ;
#4526=CARTESIAN_POINT ( 'NONE',  ( -8.993684809926110191, -9.500000000000001776, -419.2513267189134467 ) ) ;
#4527=ORIENTED_EDGE ( 'NONE', *, *, #3125, .T. ) ;
#4542=VECTOR ( 'NONE', #6823, 1000.000000000000000 ) ;
#4551=CARTESIAN_POINT ( 'NONE',  ( -26.31853765676889267, -9.500000000000001776, -432.7407288192795249 ) ) ;
#4554=DIRECTION ( 'NONE',  ( -0.9942380540931650135, 0.000000000000000000, -0.1071946444232960011 ) ) ;
#4585=DIRECTION ( 'NONE',  ( 0.4716280258120412183, 0.000000000000000000, -0.8817975988108815999 ) ) ;
#4603=LINE ( 'NONE', #3741, #4542 ) ;
#4626=DIRECTION ( 'NONE',  ( 0.000000000000000000, 1.000000000000000000, 0.000000000000000000 ) ) ;
#4635=VERTEX_POINT ( 'NONE', #3253 ) ;
#4637=AXIS2_PLACEMENT_3D ( 'NONE', #7576, #7630, #5849 ) ;
#4643=AXIS2_PLACEMENT_3D ( 'NONE', #8656, #8764, #5485 ) ;
#4665=ORIENTED_EDGE ( 'NONE', *, *, #1694, .F. ) ;
#4666=CIRCLE ( 'NONE', #1060, 15.50000000000000711 ) ;
#4679=DIRECTION ( 'NONE',  ( 0.000000000000000000, -1.000000000000000000, 0.000000000000000000 ) ) ;
#4697=CARTESIAN_POINT ( 'NONE',  ( -46.74071243419621169, -7.500000000000000888, -414.3237589990241077 ) ) ;
#4700=VECTOR ( 'NONE', #2563, 1000.000000000000000 ) ;
#4701=ORIENTED_EDGE ( 'NONE', *, *, #7615, .T. ) ;
#4723=AXIS2_PLACEMENT_3D ( 'NONE', #5674, #5624, #1652 ) ;
#4724=AXIS2_PLACEMENT_3D ( 'NONE', #5292, #359, #2881 ) ;
#4725=ORIENTED_EDGE ( 'NONE', *, *, #2683, .F. ) ;
#4731=PLANE ( 'NONE',  #767 ) ;
#4734=( GEOMETRIC_REPRESENTATION_CONTEXT ( 3 ) GLOBAL_UNCERTAINTY_ASSIGNED_CONTEXT ( ( #5168 ) ) GLOBAL_UNIT_ASSIGNED_CONTEXT ( ( #9021, #9074, #9772 ) ) REPRESENTATION_CONTEXT ( 'NONE', 'WORKASPACE' ) );
#4741=SHAPE_DEFINITION_REPRESENTATION ( #295, #1739 ) ;
#4743=DIRECTION ( 'NONE',  ( 0.1071946444232947937, 0.000000000000000000, -0.9942380540931651245 ) ) ;
#4744=DIRECTION ( 'NONE',  ( 0.000000000000000000, 1.000000000000000000, 0.000000000000000000 ) ) ;
#4763=DIRECTION ( 'NONE',  ( 0.1071946444232954182, 0.000000000000000000, -0.9942380540931651245 ) ) ;
#4770=ORIENTED_EDGE ( 'NONE', *, *, #9491, .F. ) ;
#4785=FACE_OUTER_BOUND ( 'NONE', #9875, .T. ) ;
#4801=CARTESIAN_POINT ( 'NONE',  ( -2.000000000003786749, -9.000000000000001776, -409.4999999999758415 ) ) ;
#4805=DIRECTION ( 'NONE',  ( 0.000000000000000000, 1.000000000000000000, 0.000000000000000000 ) ) ;
#4809=CIRCLE ( 'NONE', #3, 0.5000000000000004441 ) ;
#4816=CARTESIAN_POINT ( 'NONE',  ( -13.36185104352900055, -9.000000000000001776, -400.1641368440791098 ) ) ;
#4818=CIRCLE ( 'NONE', #7874, 11.99999999999997691 ) ;
#4819=ADVANCED_FACE ( 'NONE', ( #3880 ), #9624, .F. ) ;
#4832=DIRECTION ( 'NONE',  ( 0.000000000000000000, 1.000000000000000000, 0.000000000000000000 ) ) ;
#4838=EDGE_CURVE ( 'NONE', #10018, #4161, #7368, .T. ) ;
#4850=VECTOR ( 'NONE', #10464, 1000.000000000000000 ) ;
#4861=ORIENTED_EDGE ( 'NONE', *, *, #5217, .T. ) ;
#4863=VERTEX_POINT ( 'NONE', #6508 ) ;
#4867=DIRECTION ( 'NONE',  ( 0.000000000000000000, -1.000000000000000000, 0.000000000000000000 ) ) ;
#4880=CIRCLE ( 'NONE', #5730, 0.5000000000000004441 ) ;
#4883=FACE_OUTER_BOUND ( 'NONE', #7809, .T. ) ;
#4889=AXIS2_PLACEMENT_3D ( 'NONE', #10415, #7253, #8972 ) ;
#4890=AXIS2_PLACEMENT_3D ( 'NONE', #6152, #463, #7078 ) ;
#4897=CYLINDRICAL_SURFACE ( 'NONE', #7415, 12.49999999999998757 ) ;
#4906=EDGE_CURVE ( 'NONE', #7180, #6903, #2141, .T. ) ;
#4914=EDGE_LOOP ( 'NONE', ( #10318, #2058, #9814, #9399 ) ) ;
#4923=VERTEX_POINT ( 'NONE', #224 ) ;
#4932=CARTESIAN_POINT ( 'NONE',  ( -46.74071243419621169, -7.500000000000000888, -414.3237589990241077 ) ) ;
#4934=VECTOR ( 'NONE', #2144, 1000.000000000000000 ) ;
#4976=ORIENTED_EDGE ( 'NONE', *, *, #1146, .T. ) ;
#4994=DIRECTION ( 'NONE',  ( -6.262351748276267552E-13, -1.000000000000000000, 1.110223024625155531E-12 ) ) ;
#5035=DIRECTION ( 'NONE',  ( -0.5828070674935414974, 0.000000000000000000, -0.8126105599114366029 ) ) ;
#5048=COLOUR_RGB ( '', 0.31764706, 0.68627451, 0.89019608) ;
#5058=AXIS2_PLACEMENT_3D ( 'NONE', #4229, #4175, #7449 ) ;
#5083=DIRECTION ( 'NONE',  ( 0.2896000924642900820, 0.000000000000000000, 0.9571477349106952692 ) ) ;
#5097=ADVANCED_FACE ( 'NONE', ( #2042 ), #8582, .T. ) ;
#5102=CARTESIAN_POINT ( 'NONE',  ( -43.46674421124934184, -9.000000000000001776, -402.7790142173016648 ) ) ;
#5110=AXIS2_PLACEMENT_3D ( 'NONE', #6999, #10271, #5366 ) ;
#5111=FACE_OUTER_BOUND ( 'NONE', #1311, .T. ) ;
#5136=CARTESIAN_POINT ( 'NONE',  ( -27.92645732311634532, -9.000000000000001776, -417.8271580078818488 ) ) ;
#5138=MANIFOLD_SOLID_BREP ( 'Stock-MAS-686-1', #2481 ) ;
#5168=UNCERTAINTY_MEASURE_WITH_UNIT (LENGTH_MEASURE( 1.000000000000000082E-05 ), #9021, 'distance_accuracy_value', 'NONE');
#5169=DIRECTION ( 'NONE',  ( 0.000000000000000000, -1.000000000000000000, 0.000000000000000000 ) ) ;
#5171=ORIENTED_EDGE ( 'NONE', *, *, #10479, .F. ) ;
#5176=DIRECTION ( 'NONE',  ( -0.1071946444232961260, 0.000000000000000000, 0.9942380540931650135 ) ) ;
#5181=VECTOR ( 'NONE', #9561, 1000.000000000000114 ) ;
#5185=ORIENTED_EDGE ( 'NONE', *, *, #641, .T. ) ;
#5191=DIRECTION ( 'NONE',  ( 0.000000000000000000, 1.000000000000000000, 0.000000000000000000 ) ) ;
#5198=CARTESIAN_POINT ( 'NONE',  ( -19.68871134463705985, -7.500000000000000888, -416.4361005590961327 ) ) ;
#5201=ORIENTED_EDGE ( 'NONE', *, *, #6274, .T. ) ;
#5215=CIRCLE ( 'NONE', #1442, 0.5000000000000004441 ) ;
#5217=EDGE_CURVE ( 'NONE', #2675, #10018, #1825, .T. ) ;
#5258=EDGE_CURVE ( 'NONE', #3896, #10437, #4603, .T. ) ;
#5264=DIRECTION ( 'NONE',  ( -0.2728306852452879183, 0.000000000000000000, -0.9620620651437133963 ) ) ;
#5270=ORIENTED_EDGE ( 'NONE', *, *, #1160, .F. ) ;
#5274=CARTESIAN_POINT ( 'NONE',  ( -37.57635160138833896, -7.500000000000000888, -403.2777420460153053 ) ) ;
#5292=CARTESIAN_POINT ( 'NONE',  ( -39.23786858994942151, -9.000000000000001776, -387.8670522075712483 ) ) ;
#5294=( NAMED_UNIT ( * ) SI_UNIT ( $, .STERADIAN. ) SOLID_ANGLE_UNIT ( ) );
#5304=CIRCLE ( 'NONE', #8915, 12.50000000000002309 ) ;
#5349=AXIS2_PLACEMENT_3D ( 'NONE', #3053, #2361, #2303 ) ;
#5363=DIRECTION ( 'NONE',  ( 0.000000000000000000, 1.000000000000000000, 0.000000000000000000 ) ) ;
#5366=DIRECTION ( 'NONE',  ( 0.2728306852451984343, 0.000000000000000000, 0.9620620651437388204 ) ) ;
#5385=EDGE_CURVE ( 'NONE', #6619, #661, #5396, .T. ) ;
#5389=VERTEX_POINT ( 'NONE', #8926 ) ;
#5396=CIRCLE ( 'NONE', #775, 15.50000000000000711 ) ;
#5405=CARTESIAN_POINT ( 'NONE',  ( -37.45790571718422513, -8.000000000000000000, -422.6951089173222726 ) ) ;
#5406=ADVANCED_FACE ( 'NONE', ( #10591 ), #4897, .T. ) ;
#5407=ORIENTED_EDGE ( 'NONE', *, *, #184, .T. ) ;
#5428=DIRECTION ( 'NONE',  ( 1.881029090955282852E-11, 1.000000000000000000, 2.085935400224071097E-11 ) ) ;
#5442=ORIENTED_EDGE ( 'NONE', *, *, #9093, .F. ) ;
#5444=ORIENTED_EDGE ( 'NONE', *, *, #9625, .T. ) ;
#5456=ORIENTED_EDGE ( 'NONE', *, *, #10227, .F. ) ;
#5482=EDGE_CURVE ( 'NONE', #7772, #2010, #1403, .T. ) ;
#5483=CARTESIAN_POINT ( 'NONE',  ( -27.92645732311634532, -9.000000000000001776, -417.8271580078818488 ) ) ;
#5485=DIRECTION ( 'NONE',  ( 0.000000000000000000, -1.000000000000000000, 0.000000000000000000 ) ) ;
#5504=EDGE_CURVE ( 'NONE', #8504, #6903, #1581, .T. ) ;
#5506=VERTEX_POINT ( 'NONE', #2699 ) ;
#5520=CYLINDRICAL_SURFACE ( 'NONE', #4889, 12.49999999999998579 ) ;
#5528=DIRECTION ( 'NONE',  ( 0.000000000000000000, 1.000000000000000000, 0.000000000000000000 ) ) ;
#5537=ORIENTED_EDGE ( 'NONE', *, *, #8619, .F. ) ;
#5544=PLANE ( 'NONE',  #1945 ) ;
#5550=EDGE_LOOP ( 'NONE', ( #6256, #4029, #4665, #2842 ) ) ;
#5556=CIRCLE ( 'NONE', #8645, 3.500000000000020428 ) ;
#5580=VERTEX_POINT ( 'NONE', #10366 ) ;
#5598=EDGE_CURVE ( 'NONE', #2578, #7772, #6939, .T. ) ;
#5613=DIRECTION ( 'NONE',  ( 0.1071946444232947937, 0.000000000000000000, -0.9942380540931651245 ) ) ;
#5624=DIRECTION ( 'NONE',  ( 0.000000000000000000, -1.000000000000000000, 0.000000000000000000 ) ) ;
#5631=DIRECTION ( 'NONE',  ( 0.000000000000000000, 1.000000000000000000, 0.000000000000000000 ) ) ;
#5635=DIRECTION ( 'NONE',  ( 0.7426245373610527167, 0.000000000000000000, -0.6697079934637800713 ) ) ;
#5647=DIRECTION ( 'NONE',  ( -4.963222276338128250E-12, 1.000000000000000000, -2.652296088385032042E-12 ) ) ;
#5674=CARTESIAN_POINT ( 'NONE',  ( -26.31853765676889267, -7.500000000000000888, -432.7407288192795249 ) ) ;
#5701=VECTOR ( 'NONE', #533, 1000.000000000000000 ) ;
#5712=ORIENTED_EDGE ( 'NONE', *, *, #4458, .F. ) ;
#5729=DIRECTION ( 'NONE',  ( 0.1071946444232959594, 0.000000000000000000, -0.9942380540931649024 ) ) ;
#5730=AXIS2_PLACEMENT_3D ( 'NONE', #5912, #7634, #5852 ) ;
#5751=DIRECTION ( 'NONE',  ( -0.1071946444232964035, 0.000000000000000000, 0.9942380540931649024 ) ) ;
#5775=DIRECTION ( 'NONE',  ( -0.1071946444232954182, 0.000000000000000000, 0.9942380540931651245 ) ) ;
#5783=CARTESIAN_POINT ( 'NONE',  ( -2.000000000003786749, -9.000000000000001776, -409.4999999999758415 ) ) ;
#5786=DIRECTION ( 'NONE',  ( 0.000000000000000000, 1.000000000000000000, 0.000000000000000000 ) ) ;
#5792=ORIENTED_EDGE ( 'NONE', *, *, #1203, .F. ) ;
#5800=EDGE_CURVE ( 'NONE', #4863, #2810, #7923, .T. ) ;
#5805=ORIENTED_EDGE ( 'NONE', *, *, #9172, .F. ) ;
#5818=CIRCLE ( 'NONE', #3761, 0.5000000000000004441 ) ;
#5831=CARTESIAN_POINT ( 'NONE',  ( -3.339933055294988851, -8.000000000000000000, -397.0720243238112630 ) ) ;
#5840=DIRECTION ( 'NONE',  ( 0.5828070674935411644, 0.000000000000000000, 0.8126105599114369360 ) ) ;
#5841=CARTESIAN_POINT ( 'NONE',  ( -13.36185104352900055, -9.000000000000001776, -400.1641368440791098 ) ) ;
#5849=DIRECTION ( 'NONE',  ( -0.2728306852451987119, 0.000000000000000000, -0.9620620651437387094 ) ) ;
#5852=DIRECTION ( 'NONE',  ( 0.000000000000000000, -1.000000000000000000, 0.000000000000000000 ) ) ;
#5862=CARTESIAN_POINT ( 'NONE',  ( -19.68871134463705985, -9.500000000000001776, -416.4361005590961327 ) ) ;
#5867=DIRECTION ( 'NONE',  ( 0.1071946444232958900, 0.000000000000000000, -0.9942380540931649024 ) ) ;
#5890=PRESENTATION_STYLE_ASSIGNMENT (( #2626 ) ) ;
#5893=DIRECTION ( 'NONE',  ( 0.000000000000000000, -1.000000000000000000, 0.000000000000000000 ) ) ;
#5899=ORIENTED_EDGE ( 'NONE', *, *, #8111, .F. ) ;
#5912=CARTESIAN_POINT ( 'NONE',  ( -37.57635160138833896, -9.000000000000001776, -403.2777420460153053 ) ) ;
#5921=UNCERTAINTY_MEASURE_WITH_UNIT (LENGTH_MEASURE( 1.000000000000000082E-05 ), #9665, 'distance_accuracy_value', 'NONE');
#5931=( GEOMETRIC_REPRESENTATION_CONTEXT ( 3 ) GLOBAL_UNCERTAINTY_ASSIGNED_CONTEXT ( ( #4102 ) ) GLOBAL_UNIT_ASSIGNED_CONTEXT ( ( #6052, #9240, #5294 ) ) REPRESENTATION_CONTEXT ( 'NONE', 'WORKASPACE' ) );
#5947=CARTESIAN_POINT ( 'NONE',  ( -46.74071243419621169, -9.500000000000001776, -414.3237589990241077 ) ) ;
#5948=LINE ( 'NONE', #5136, #1888 ) ;
#5957=VERTEX_POINT ( 'NONE', #9300 ) ;
#5963=DIRECTION ( 'NONE',  ( 0.9942380540931650135, 0.000000000000000000, 0.1071946444232960011 ) ) ;
#5974=LINE ( 'NONE', #8285, #1183 ) ;
#5980=ORIENTED_EDGE ( 'NONE', *, *, #1426, .F. ) ;
#5985=LINE ( 'NONE', #8762, #2580 ) ;
#5994=FACE_OUTER_BOUND ( 'NONE', #5550, .T. ) ;
#6020=DIRECTION ( 'NONE',  ( -0.7494507079133034821, 0.000000000000000000, 0.6620601456123518247 ) ) ;
#6021=EDGE_CURVE ( 'NONE', #911, #2578, #4666, .T. ) ;
#6029=CARTESIAN_POINT ( 'NONE',  ( -13.36185104356876785, -8.000000000000000000, -400.1641368440833730 ) ) ;
#6030=DIRECTION ( 'NONE',  ( 0.000000000000000000, -1.000000000000000000, 0.000000000000000000 ) ) ;
#6046=DIRECTION ( 'NONE',  ( 0.000000000000000000, 1.000000000000000000, 0.000000000000000000 ) ) ;
#6052=( LENGTH_UNIT ( ) NAMED_UNIT ( * ) SI_UNIT ( .MILLI., .METRE. ) );
#6058=EDGE_LOOP ( 'NONE', ( #4770, #2866, #905, #764 ) ) ;
#6059=DIRECTION ( 'NONE',  ( -0.7426245373609573486, 0.000000000000000000, 0.6697079934638857646 ) ) ;
#6060=ORIENTED_EDGE ( 'NONE', *, *, #4489, .T. ) ;
#6069=LINE ( 'NONE', #10216, #6775 ) ;
#6079=DIRECTION ( 'NONE',  ( 0.9942380540931650135, 0.000000000000000000, 0.1071946444232960011 ) ) ;
#6082=EDGE_CURVE ( 'NONE', #4372, #4635, #3683, .T. ) ;
#6090=DIRECTION ( 'NONE',  ( 0.9942380540931649024, 0.000000000000000000, 0.1071946444232959872 ) ) ;
#6136=CYLINDRICAL_SURFACE ( 'NONE', #1411, 12.49999999999998579 ) ;
#6143=ORIENTED_EDGE ( 'NONE', *, *, #4174, .F. ) ;
#6152=CARTESIAN_POINT ( 'NONE',  ( -14.96977070983867009, -9.633703999999999823, -385.2505660326773409 ) ) ;
#6165=DIRECTION ( 'NONE',  ( 0.000000000000000000, -1.000000000000000000, 0.000000000000000000 ) ) ;
#6167=CIRCLE ( 'NONE', #692, 0.5000000000000004441 ) ;
#6170=DIRECTION ( 'NONE',  ( 0.000000000000000000, 1.000000000000000000, 0.000000000000000000 ) ) ;
#6179=CARTESIAN_POINT ( 'NONE',  ( -2.000000000003786749, -9.500000000000001776, -409.4999999999758415 ) ) ;
#6192=ORIENTED_EDGE ( 'NONE', *, *, #7629, .F. ) ;
#6193=CARTESIAN_POINT ( 'NONE',  ( -14.96977070983867009, -9.500000000000001776, -385.2505660326773409 ) ) ;
#6200=FACE_OUTER_BOUND ( 'NONE', #6607, .T. ) ;
#6208=AXIS2_PLACEMENT_3D ( 'NONE', #1038, #4162, #1690 ) ;
#6214=ORIENTED_EDGE ( 'NONE', *, *, #7921, .F. ) ;
#6219=CARTESIAN_POINT ( 'NONE',  ( -9.285088343770869557, -9.000000000000001776, -419.6576319987959778 ) ) ;
#6252=CIRCLE ( 'NONE', #9009, 15.00000000000002309 ) ;
#6256=ORIENTED_EDGE ( 'NONE', *, *, #1160, .T. ) ;
#6274=EDGE_CURVE ( 'NONE', #5389, #5957, #7424, .T. ) ;
#6299=AXIS2_PLACEMENT_3D ( 'NONE', #10010, #282, #8439 ) ;
#6324=SURFACE_STYLE_USAGE ( .BOTH. , #3056 ) ;
#6328=AXIS2_PLACEMENT_3D ( 'NONE', #6652, #6597, #5083 ) ;
#6329=AXIS2_PLACEMENT_3D ( 'NONE', #1486, #4867, #4763 ) ;
#6331=APPLICATION_CONTEXT ( 'automotive_design' ) ;
#6359=ADVANCED_FACE ( 'NONE', ( #2606 ), #134, .F. ) ;
#6381=CYLINDRICAL_SURFACE ( 'NONE', #1243, 3.500000000000020428 ) ;
#6399=ADVANCED_FACE ( 'NONE', ( #8503 ), #6136, .T. ) ;
#6412=ORIENTED_EDGE ( 'NONE', *, *, #8864, .F. ) ;
#6421=CARTESIAN_POINT ( 'NONE',  ( -26.31853765676889267, -8.000000000000000000, -432.7407288192795249 ) ) ;
#6458=ORIENTED_EDGE ( 'NONE', *, *, #6021, .T. ) ;
#6496=DIRECTION ( 'NONE',  ( -0.1071946444232959872, 0.000000000000000000, 0.9942380540931649024 ) ) ;
#6498=( NAMED_UNIT ( * ) SI_UNIT ( $, .STERADIAN. ) SOLID_ANGLE_UNIT ( ) );
#6502=ORIENTED_EDGE ( 'NONE', *, *, #3536, .T. ) ;
#6508=CARTESIAN_POINT ( 'NONE',  ( -2.375181255485324439, -7.500000000000000888, -406.0201668106497550 ) ) ;
#6522=ORIENTED_EDGE ( 'NONE', *, *, #4366, .F. ) ;
#6553=VERTEX_POINT ( 'NONE', #343 ) ;
#6562=CIRCLE ( 'NONE', #4336, 12.00000000000001243 ) ;
#6565=AXIS2_PLACEMENT_3D ( 'NONE', #5783, #3381, #5035 ) ;
#6567=EDGE_LOOP ( 'NONE', ( #9804, #4976 ) ) ;
#6572=AXIS2_PLACEMENT_3D ( 'NONE', #7514, #8320, #5840 ) ;
#6585=EDGE_CURVE ( 'NONE', #2010, #6619, #6562, .T. ) ;
#6593=VERTEX_POINT ( 'NONE', #4325 ) ;
#6597=DIRECTION ( 'NONE',  ( 0.000000000000000000, 1.000000000000000000, 0.000000000000000000 ) ) ;
#6607=EDGE_LOOP ( 'NONE', ( #4725, #3169, #6502, #4015 ) ) ;
#6610=AXIS2_PLACEMENT_3D ( 'NONE', #4091, #1462, #4743 ) ;
#6612=ORIENTED_EDGE ( 'NONE', *, *, #9605, .F. ) ;
#6618=CARTESIAN_POINT ( 'NONE',  ( -37.57635160138833896, -8.000000000000000000, -403.2777420460153053 ) ) ;
#6619=VERTEX_POINT ( 'NONE', #10170 ) ;
#6630=DIRECTION ( 'NONE',  ( -0.9942380540931649024, 0.000000000000000000, -0.1071946444232959872 ) ) ;
#6648=VERTEX_POINT ( 'NONE', #5274 ) ;
#6652=CARTESIAN_POINT ( 'NONE',  ( -46.74071243419621169, -9.000000000000001776, -414.3237589990241077 ) ) ;
#6657=CIRCLE ( 'NONE', #3564, 11.99999999999999289 ) ;
#6660=PRODUCT_DEFINITION ( 'UNKNOWN', '', #4405, #4417 ) ;
#6690=DIRECTION ( 'NONE',  ( 0.9620620651437388204, -2.527616691482515415E-15, -0.2728306852451987674 ) ) ;
#6710=DIRECTION ( 'NONE',  ( 0.1071946444232958900, 0.000000000000000000, -0.9942380540931649024 ) ) ;
#6730=DIRECTION ( 'NONE',  ( 0.000000000000000000, 1.000000000000000000, 0.000000000000000000 ) ) ;
#6736=EDGE_CURVE ( 'NONE', #7240, #8504, #4818, .T. ) ;
#6737=CARTESIAN_POINT ( 'NONE',  ( -37.72923359849013281, -8.000000000000000000, -403.2942251520989316 ) ) ;
#6742=ORIENTED_EDGE ( 'NONE', *, *, #9491, .T. ) ;
#6746=CARTESIAN_POINT ( 'NONE',  ( -39.23786858994942151, -9.633703999999999823, -387.8670522075712483 ) ) ;
#6761=FACE_OUTER_BOUND ( 'NONE', #2122, .T. ) ;
#6775=VECTOR ( 'NONE', #2852, 1000.000000000000000 ) ;
#6789=DIRECTION ( 'NONE',  ( -0.7426245373610013134, 0.000000000000000000, 0.6697079934638370258 ) ) ;
#6794=DIRECTION ( 'NONE',  ( 0.2728306852451984343, 0.000000000000000000, 0.9620620651437388204 ) ) ;
#6806=ORIENTED_EDGE ( 'NONE', *, *, #6585, .T. ) ;
#6808=ADVANCED_FACE ( 'NONE', ( #7092 ), #7562, .T. ) ;
#6816=TOROIDAL_SURFACE ( 'NONE', #8183, 15.50000000000000000, 0.5000000000000000000 ) ;
#6823=DIRECTION ( 'NONE',  ( 0.000000000000000000, 1.000000000000000000, 0.000000000000000000 ) ) ;
#6841=CARTESIAN_POINT ( 'NONE',  ( -39.23786858994942151, -7.500000000000000888, -387.8670522075712483 ) ) ;
#6843=CYLINDRICAL_SURFACE ( 'NONE', #2544, 0.5000000000000004441 ) ;
#6848=ORIENTED_EDGE ( 'NONE', *, *, #7668, .F. ) ;
#6871=FILL_AREA_STYLE ('',( #410 ) ) ;
#6877=ORIENTED_EDGE ( 'NONE', *, *, #6967, .T. ) ;
#6881=CIRCLE ( 'NONE', #179, 0.5000000000000004441 ) ;
#6889=CARTESIAN_POINT ( 'NONE',  ( -46.74071243419621169, -8.000000000000000000, -414.3237589990241077 ) ) ;
#6900=CARTESIAN_POINT ( 'NONE',  ( -37.62994892356022092, -9.000000000000001776, -402.7806230189644339 ) ) ;
#6903=VERTEX_POINT ( 'NONE', #1026 ) ;
#6915=VERTEX_POINT ( 'NONE', #5405 ) ;
#6922=SURFACE_STYLE_FILL_AREA ( #6871 ) ;
#6923=CARTESIAN_POINT ( 'NONE',  ( -45.40077937890500692, -9.000000000000001776, -426.7517346751886862 ) ) ;
#6939=LINE ( 'NONE', #8748, #5181 ) ;
#6940=EDGE_CURVE ( 'NONE', #661, #2675, #3779, .T. ) ;
#6949=AXIS2_PLACEMENT_3D ( 'NONE', #7783, #801, #2307 ) ;
#6967=EDGE_CURVE ( 'NONE', #10131, #10253, #2740, .T. ) ;
#6976=DIRECTION ( 'NONE',  ( 0.000000000000000000, -1.000000000000000000, 0.000000000000000000 ) ) ;
#6985=CARTESIAN_POINT ( 'NONE',  ( -13.30825372127758399, -9.000000000000001776, -400.6612558711213410 ) ) ;
#6988=CARTESIAN_POINT ( 'NONE',  ( -46.74071243419621169, -9.000000000000001776, -414.3237589990241077 ) ) ;
#6999=CARTESIAN_POINT ( 'NONE',  ( -46.74071243419621169, -9.000000000000001776, -414.3237589990241077 ) ) ;
#7009=EDGE_LOOP ( 'NONE', ( #9858, #7310, #620, #5712 ) ) ;
#7041=DIRECTION ( 'NONE',  ( 0.000000000000000000, -1.000000000000000000, 0.000000000000000000 ) ) ;
#7042=AXIS2_PLACEMENT_3D ( 'NONE', #4025, #4832, #6496 ) ;
#7049=DIRECTION ( 'NONE',  ( 0.000000000000000000, 1.000000000000000000, 0.000000000000000000 ) ) ;
#7054=EDGE_CURVE ( 'NONE', #9639, #1033, #8728, .T. ) ;
#7069=VERTEX_POINT ( 'NONE', #844 ) ;
#7078=DIRECTION ( 'NONE',  ( 0.4716280258120412183, 0.000000000000000000, -0.8817975988108815999 ) ) ;
#7089=ORIENTED_EDGE ( 'NONE', *, *, #7629, .T. ) ;
#7092=FACE_OUTER_BOUND ( 'NONE', #2401, .T. ) ;
#7118=CARTESIAN_POINT ( 'NONE',  ( -41.12300563599592351, -9.500000000000001776, -403.1572299801428017 ) ) ;
#7167=CYLINDRICAL_SURFACE ( 'NONE', #1678, 12.49999999999998579 ) ;
#7179=VECTOR ( 'NONE', #6976, 1000.000000000000000 ) ;
#7180=VERTEX_POINT ( 'NONE', #9716 ) ;
#7193=ORIENTED_EDGE ( 'NONE', *, *, #7851, .T. ) ;
#7203=CIRCLE ( 'NONE', #4452, 3.500000000000020428 ) ;
#7208=VECTOR ( 'NONE', #7902, 1000.000000000000114 ) ;
#7226=ORIENTED_EDGE ( 'NONE', *, *, #1880, .T. ) ;
#7230=EDGE_LOOP ( 'NONE', ( #7193, #3723, #8448, #4701, #6214, #5899 ) ) ;
#7239=DIRECTION ( 'NONE',  ( -0.5828070674935414974, 0.000000000000000000, -0.8126105599114366029 ) ) ;
#7240=VERTEX_POINT ( 'NONE', #8257 ) ;
#7251=DIRECTION ( 'NONE',  ( -0.09270529807100655328, 0.000000000000000000, 0.9956935912767369556 ) ) ;
#7253=DIRECTION ( 'NONE',  ( 0.000000000000000000, 1.000000000000000000, 0.000000000000000000 ) ) ;
#7254=ORIENTED_EDGE ( 'NONE', *, *, #2346, .F. ) ;
#7259=CIRCLE ( 'NONE', #7427, 3.500000000000020428 ) ;
#7265=ADVANCED_FACE ( 'NONE', ( #950 ), #3599, .T. ) ;
#7275=ADVANCED_FACE ( 'NONE', ( #8363 ), #4181, .F. ) ;
#7288=VECTOR ( 'NONE', #8588, 1000.000000000000114 ) ;
#7300=DIRECTION ( 'NONE',  ( 0.000000000000000000, 1.000000000000000000, 0.000000000000000000 ) ) ;
#7308=DIRECTION ( 'NONE',  ( 0.000000000000000000, -1.000000000000000000, 0.000000000000000000 ) ) ;
#7309=EDGE_CURVE ( 'NONE', #4372, #1489, #335, .T. ) ;
#7310=ORIENTED_EDGE ( 'NONE', *, *, #2013, .F. ) ;
#7334=ORIENTED_EDGE ( 'NONE', *, *, #7668, .T. ) ;
#7339=EDGE_CURVE ( 'NONE', #3077, #7180, #668, .T. ) ;
#7345=ORIENTED_EDGE ( 'NONE', *, *, #3536, .F. ) ;
#7348=EDGE_LOOP ( 'NONE', ( #9471, #8287, #6192, #6522 ) ) ;
#7362=ORIENTED_EDGE ( 'NONE', *, *, #8616, .F. ) ;
#7368=LINE ( 'NONE', #3932, #7975 ) ;
#7400=ORIENTED_EDGE ( 'NONE', *, *, #3321, .T. ) ;
#7415=AXIS2_PLACEMENT_3D ( 'NONE', #3343, #7863, #5751 ) ;
#7424=CIRCLE ( 'NONE', #6208, 3.500000000000020428 ) ;
#7427=AXIS2_PLACEMENT_3D ( 'NONE', #6179, #10273, #2910 ) ;
#7441=ORIENTED_EDGE ( 'NONE', *, *, #8921, .T. ) ;
#7449=DIRECTION ( 'NONE',  ( 0.1071946444232959594, 0.000000000000000000, -0.9942380540931649024 ) ) ;
#7485=EDGE_CURVE ( 'NONE', #5506, #10253, #9637, .T. ) ;
#7514=CARTESIAN_POINT ( 'NONE',  ( -18.02719435607597021, -7.500000000000000888, -431.8467903975401896 ) ) ;
#7525=DIRECTION ( 'NONE',  ( 6.938893903907222067E-14, -1.000000000000000000, -1.110223024625155531E-13 ) ) ;
#7532=EDGE_LOOP ( 'NONE', ( #8527, #4861, #6412, #8359 ) ) ;
#7539=ORIENTED_EDGE ( 'NONE', *, *, #4174, .T. ) ;
#7551=AXIS2_PLACEMENT_3D ( 'NONE', #3751, #7041, #4455 ) ;
#7562=TOROIDAL_SURFACE ( 'NONE', #2923, 15.50000000000000000, 0.5000000000000000000 ) ;
#7576=CARTESIAN_POINT ( 'NONE',  ( -39.23786858994942151, -8.000000000000000000, -387.8670522075712483 ) ) ;
#7595=EDGE_LOOP ( 'NONE', ( #2404, #647, #10557, #3407 ) ) ;
#7596=DIRECTION ( 'NONE',  ( 0.000000000000000000, 1.000000000000000000, 0.000000000000000000 ) ) ;
#7598=LINE ( 'NONE', #2059, #1269 ) ;
#7608=ORIENTED_EDGE ( 'NONE', *, *, #10479, .T. ) ;
#7615=EDGE_CURVE ( 'NONE', #3896, #2293, #5304, .T. ) ;
#7629=EDGE_CURVE ( 'NONE', #4350, #4635, #2226, .T. ) ;
#7630=DIRECTION ( 'NONE',  ( 0.000000000000000000, -1.000000000000000000, 0.000000000000000000 ) ) ;
#7634=DIRECTION ( 'NONE',  ( -0.9942380540931650135, 0.000000000000000000, -0.1071946444232960011 ) ) ;
#7644=DIRECTION ( 'NONE',  ( 0.000000000000000000, 1.000000000000000000, 0.000000000000000000 ) ) ;
#7660=ORIENTED_EDGE ( 'NONE', *, *, #1694, .T. ) ;
#7668=EDGE_CURVE ( 'NONE', #4635, #7069, #5974, .T. ) ;
#7690=DIRECTION ( 'NONE',  ( 0.9942380540931650135, 0.000000000000000000, 0.1071946444232960011 ) ) ;
#7736=DIRECTION ( 'NONE',  ( 0.000000000000000000, 1.000000000000000000, 0.000000000000000000 ) ) ;
#7772=VERTEX_POINT ( 'NONE', #5862 ) ;
#7777=AXIS2_PLACEMENT_3D ( 'NONE', #2022, #2775, #4392 ) ;
#7783=CARTESIAN_POINT ( 'NONE',  ( -13.09107633769369095, -9.000000000000001776, -400.6378407017721202 ) ) ;
#7785=VECTOR ( 'NONE', #3933, 1000.000000000000114 ) ;
#7809=EDGE_LOOP ( 'NONE', ( #1382, #6143, #398, #7608 ) ) ;
#7828=DIRECTION ( 'NONE',  ( 0.000000000000000000, -1.000000000000000000, 0.000000000000000000 ) ) ;
#7829=CIRCLE ( 'NONE', #9222, 0.5000000000000004441 ) ;
#7838=FACE_OUTER_BOUND ( 'NONE', #10015, .T. ) ;
#7847=CARTESIAN_POINT ( 'NONE',  ( -27.98005464532998232, -8.000000000000000000, -417.3300389808354680 ) ) ;
#7851=EDGE_CURVE ( 'NONE', #1033, #6553, #3081, .T. ) ;
#7863=DIRECTION ( 'NONE',  ( 0.000000000000000000, 1.000000000000000000, 0.000000000000000000 ) ) ;
#7874=AXIS2_PLACEMENT_3D ( 'NONE', #8126, #6730, #814 ) ;
#7887=AXIS2_PLACEMENT_3D ( 'NONE', #5102, #222, #9201 ) ;
#7902=DIRECTION ( 'NONE',  ( 0.9942380540931649024, 0.000000000000000000, 0.1071946444232959872 ) ) ;
#7908=CARTESIAN_POINT ( 'NONE',  ( -7.895350322666780940, -9.000000000000001776, -398.4775300148504016 ) ) ;
#7909=EDGE_CURVE ( 'NONE', #6619, #9376, #6881, .T. ) ;
#7911=EDGE_CURVE ( 'NONE', #168, #4161, #8406, .T. ) ;
#7921=EDGE_CURVE ( 'NONE', #911, #2293, #4809, .T. ) ;
#7923=CIRCLE ( 'NONE', #39, 3.500000000000020428 ) ;
#7931=ORIENTED_EDGE ( 'NONE', *, *, #184, .F. ) ;
#7939=EDGE_CURVE ( 'NONE', #24, #6915, #8919, .T. ) ;
#7940=CIRCLE ( 'NONE', #3313, 3.500000000000020428 ) ;
#7941=ORIENTED_EDGE ( 'NONE', *, *, #554, .T. ) ;
#7943=DIRECTION ( 'NONE',  ( 4.270328125766856294E-11, 1.000000000000000000, -3.062867458902624639E-11 ) ) ;
#7948=DIRECTION ( 'NONE',  ( 0.7426245373610016465, 0.000000000000000000, -0.6697079934638365817 ) ) ;
#7954=EDGE_CURVE ( 'NONE', #6648, #4161, #6167, .T. ) ;
#7975=VECTOR ( 'NONE', #2376, 1000.000000000000000 ) ;
#7976=ORIENTED_EDGE ( 'NONE', *, *, #4906, .F. ) ;
#8015=LINE ( 'NONE', #2482, #7785 ) ;
#8030=ORIENTED_EDGE ( 'NONE', *, *, #6082, .T. ) ;
#8040=EDGE_LOOP ( 'NONE', ( #4419, #6877, #2641, #9749, #2327, #2296 ) ) ;
#8043=DIRECTION ( 'NONE',  ( 0.000000000000000000, 1.000000000000000000, 0.000000000000000000 ) ) ;
#8048=DIRECTION ( 'NONE',  ( 0.1071946444232947937, 0.000000000000000000, -0.9942380540931651245 ) ) ;
#8049=CARTESIAN_POINT ( 'NONE',  ( -12.57072393360216722, -9.500000000000001776, -416.1715661968751192 ) ) ;
#8103=AXIS2_PLACEMENT_3D ( 'NONE', #104, #9241, #3541 ) ;
#8111=EDGE_CURVE ( 'NONE', #1033, #911, #3946, .T. ) ;
#8126=CARTESIAN_POINT ( 'NONE',  ( -2.000000000003786749, -7.500000000000000888, -409.4999999999758415 ) ) ;
#8130=AXIS2_PLACEMENT_3D ( 'NONE', #5947, #3534, #2726 ) ;
#8135=FACE_OUTER_BOUND ( 'NONE', #739, .T. ) ;
#8138=TOROIDAL_SURFACE ( 'NONE', #9860, 15.50000000000000000, 0.5000000000000000000 ) ;
#8147=AXIS2_PLACEMENT_3D ( 'NONE', #6421, #882, #9706 ) ;
#8150=EDGE_LOOP ( 'NONE', ( #2436, #2501, #1971, #7976 ) ) ;
#8161=DIRECTION ( 'NONE',  ( 0.000000000000000000, -1.000000000000000000, 0.000000000000000000 ) ) ;
#8166=EDGE_LOOP ( 'NONE', ( #1861, #10347, #3438, #9027 ) ) ;
#8169=ADVANCED_FACE ( 'NONE', ( #3703, #1611, #9557 ), #10518, .F. ) ;
#8172=ADVANCED_FACE ( 'NONE', ( #697 ), #2415, .T. ) ;
#8183=AXIS2_PLACEMENT_3D ( 'NONE', #9262, #280, #6020 ) ;
#8207=CARTESIAN_POINT ( 'NONE',  ( -39.23786858994942151, -9.500000000000001776, -387.8670522075712483 ) ) ;
#8209=FACE_OUTER_BOUND ( 'NONE', #9218, .T. ) ;
#8211=FACE_OUTER_BOUND ( 'NONE', #1342, .T. ) ;
#8238=ORIENTED_EDGE ( 'NONE', *, *, #5800, .F. ) ;
#8254=CARTESIAN_POINT ( 'NONE',  ( -2.000000000003786749, -8.000000000000000000, -409.4999999999758415 ) ) ;
#8257=CARTESIAN_POINT ( 'NONE',  ( -7.659536309752155603, -7.500000000000000888, -398.9184288142485570 ) ) ;
#8263=CARTESIAN_POINT ( 'NONE',  ( -19.63511402242740189, -9.000000000000001776, -416.9332195861429113 ) ) ;
#8274=CARTESIAN_POINT ( 'NONE',  ( -7.659536309752155603, -9.000000000000001776, -398.9184288142485570 ) ) ;
#8277=CARTESIAN_POINT ( 'NONE',  ( -8.993684809926110191, -8.000000000000000000, -419.2513267189134467 ) ) ;
#8279=CIRCLE ( 'NONE', #8103, 12.50000000000001243 ) ;
#8281=CARTESIAN_POINT ( 'NONE',  ( -37.82921798586438911, -7.500000000000000888, -422.3602549205895684 ) ) ;
#8285=CARTESIAN_POINT ( 'NONE',  ( -19.63511402242640713, -8.000000000000000000, -416.9332195861427977 ) ) ;
#8287=ORIENTED_EDGE ( 'NONE', *, *, #9172, .T. ) ;
#8291=ORIENTED_EDGE ( 'NONE', *, *, #8864, .T. ) ;
#8307=CYLINDRICAL_SURFACE ( 'NONE', #8466, 0.5000000000000004441 ) ;
#8320=DIRECTION ( 'NONE',  ( 0.000000000000000000, -1.000000000000000000, 0.000000000000000000 ) ) ;
#8340=FACE_OUTER_BOUND ( 'NONE', #7348, .T. ) ;
#8359=ORIENTED_EDGE ( 'NONE', *, *, #1195, .F. ) ;
#8361=DIRECTION ( 'NONE',  ( 0.000000000000000000, -1.000000000000000000, 0.000000000000000000 ) ) ;
#8363=FACE_OUTER_BOUND ( 'NONE', #9208, .T. ) ;
#8382=DIRECTION ( 'NONE',  ( 0.6697079934638360266, -2.513318893526203994E-16, 0.7426245373610022016 ) ) ;
#8398=ORIENTED_EDGE ( 'NONE', *, *, #6967, .F. ) ;
#8401=DIRECTION ( 'NONE',  ( 0.000000000000000000, -1.000000000000000000, 0.000000000000000000 ) ) ;
#8406=CIRCLE ( 'NONE', #4637, 15.00000000000000711 ) ;
#8430=ORIENTED_EDGE ( 'NONE', *, *, #7615, .F. ) ;
#8439=DIRECTION ( 'NONE',  ( 0.5945784143118931775, 0.000000000000000000, 0.8040376292402952041 ) ) ;
#8448=ORIENTED_EDGE ( 'NONE', *, *, #2346, .T. ) ;
#8466=AXIS2_PLACEMENT_3D ( 'NONE', #4179, #9286, #8361 ) ;
#8503=FACE_OUTER_BOUND ( 'NONE', #6058, .T. ) ;
#8504=VERTEX_POINT ( 'NONE', #3417 ) ;
#8527=ORIENTED_EDGE ( 'NONE', *, *, #6940, .T. ) ;
#8535=DIRECTION ( 'NONE',  ( 0.000000000000000000, 1.000000000000000000, 0.000000000000000000 ) ) ;
#8538=DIRECTION ( 'NONE',  ( 0.000000000000000000, 1.000000000000000000, 0.000000000000000000 ) ) ;
#8541=CARTESIAN_POINT ( 'NONE',  ( -37.45790571715708239, -9.000000000000001776, -422.6951089172942488 ) ) ;
#8542=CARTESIAN_POINT ( 'NONE',  ( -0.6600669447125837586, -9.000000000000001776, -421.9279756761403632 ) ) ;
#8551=CARTESIAN_POINT ( 'NONE',  ( -2.000000000003786749, -7.500000000000000888, -409.4999999999758415 ) ) ;
#8562=CARTESIAN_POINT ( 'NONE',  ( -39.23786858994942151, -9.000000000000001776, -387.8670522075712483 ) ) ;
#8563=CARTESIAN_POINT ( 'NONE',  ( -46.74071243419621169, -9.500000000000001776, -414.3237589990241077 ) ) ;
#8582=CYLINDRICAL_SURFACE ( 'NONE', #6949, 0.5000000000000004441 ) ;
#8588=DIRECTION ( 'NONE',  ( -0.9942380540931625710, 0.000000000000000000, -0.1071946444233179835 ) ) ;
#8590=CARTESIAN_POINT ( 'NONE',  ( -2.375181255485324439, -9.500000000000001776, -406.0201668106497550 ) ) ;
#8610=EDGE_LOOP ( 'NONE', ( #3517, #7362, #2648, #6848 ) ) ;
#8616=EDGE_CURVE ( 'NONE', #830, #4372, #3766, .T. ) ;
#8619=EDGE_CURVE ( 'NONE', #2293, #6915, #5985, .T. ) ;
#8633=CARTESIAN_POINT ( 'NONE',  ( -47.11589368967775471, -9.500000000000001776, -410.8439258096980780 ) ) ;
#8634=CARTESIAN_POINT ( 'NONE',  ( 0.000000000000000000, 0.000000000000000000, 0.000000000000000000 ) ) ;
#8645=AXIS2_PLACEMENT_3D ( 'NONE', #8551, #8401, #4327 ) ;
#8649=CIRCLE ( 'NONE', #10546, 0.5000000000000004441 ) ;
#8650=DIRECTION ( 'NONE',  ( -0.9942380540931650135, 0.000000000000000000, -0.1071946444232960011 ) ) ;
#8656=CARTESIAN_POINT ( 'NONE',  ( -19.68871134463705985, -9.000000000000001776, -416.4361005590961327 ) ) ;
#8662=CARTESIAN_POINT ( 'NONE',  ( -14.96977070983867009, -8.000000000000000000, -385.2505660326773409 ) ) ;
#8665=ORIENTED_EDGE ( 'NONE', *, *, #5482, .T. ) ;
#8675=LINE ( 'NONE', #1265, #7179 ) ;
#8681=ORIENTED_EDGE ( 'NONE', *, *, #9093, .T. ) ;
#8713=DIRECTION ( 'NONE',  ( 0.000000000000000000, 1.000000000000000000, 0.000000000000000000 ) ) ;
#8728=CIRCLE ( 'NONE', #4111, 15.50000000000001421 ) ;
#8737=DIRECTION ( 'NONE',  ( -0.2868111944991166840, 0.000000000000000000, -0.9579871286765756500 ) ) ;
#8748=CARTESIAN_POINT ( 'NONE',  ( -27.98005464532998232, -9.500000000000001776, -417.3300389808354680 ) ) ;
#8750=ADVANCED_FACE ( 'NONE', ( #3232 ), #8138, .T. ) ;
#8756=EDGE_CURVE ( 'NONE', #4350, #6593, #8015, .T. ) ;
#8762=CARTESIAN_POINT ( 'NONE',  ( -37.45790571715708239, -9.000000000000001776, -422.6951089172942488 ) ) ;
#8764=DIRECTION ( 'NONE',  ( 0.9942380540931650135, 0.000000000000000000, 0.1071946444232960011 ) ) ;
#8768=DIRECTION ( 'NONE',  ( -0.5828070674935414974, 0.000000000000000000, -0.8126105599114366029 ) ) ;
#8769=AXIS2_PLACEMENT_3D ( 'NONE', #8662, #2169, #10236 ) ;
#8775=EDGE_LOOP ( 'NONE', ( #671, #9232, #3532, #6458, #3666, #8665, #6806, #3290 ) ) ;
#8777=ORIENTED_EDGE ( 'NONE', *, *, #7911, .F. ) ;
#8786=EDGE_LOOP ( 'NONE', ( #2789, #7931, #10200, #8838 ) ) ;
#8789=TOROIDAL_SURFACE ( 'NONE', #5349, 12.00000000000000000, 0.5000000000000000000 ) ;
#8803=FACE_BOUND ( 'NONE', #6567, .T. ) ;
#8811=CIRCLE ( 'NONE', #4195, 15.00000000000001776 ) ;
#8826=AXIS2_PLACEMENT_3D ( 'NONE', #3431, #5893, #6710 ) ;
#8838=ORIENTED_EDGE ( 'NONE', *, *, #4489, .F. ) ;
#8841=ADVANCED_FACE ( 'NONE', ( #10590 ), #1788, .T. ) ;
#8854=DIRECTION ( 'NONE',  ( -0.4716280258120416069, 0.000000000000000000, 0.8817975988108813779 ) ) ;
#8861=CARTESIAN_POINT ( 'NONE',  ( -24.37035621709999944, -7.500000000000000888, -411.9118794995000030 ) ) ;
#8863=DIRECTION ( 'NONE',  ( -0.1071946444232954182, 0.000000000000000000, 0.9942380540931651245 ) ) ;
#8864=EDGE_CURVE ( 'NONE', #9639, #10018, #4880, .T. ) ;
#8875=DIRECTION ( 'NONE',  ( 0.000000000000000000, 1.000000000000000000, 0.000000000000000000 ) ) ;
#8889=ORIENTED_EDGE ( 'NONE', *, *, #7939, .T. ) ;
#8915=AXIS2_PLACEMENT_3D ( 'NONE', #3512, #5169, #6794 ) ;
#8918=CARTESIAN_POINT ( 'NONE',  ( -46.74071243419621169, -7.500000000000000888, -414.3237589990241077 ) ) ;
#8919=CIRCLE ( 'NONE', #346, 0.5000000000000004441 ) ;
#8921=EDGE_CURVE ( 'NONE', #6648, #10492, #10105, .T. ) ;
#8926=CARTESIAN_POINT ( 'NONE',  ( -46.36553117871467578, -7.500000000000000888, -417.8035921883502510 ) ) ;
#8950=ADVANCED_FACE ( 'NONE', ( #7838 ), #173, .T. ) ;
#8959=CARTESIAN_POINT ( 'NONE',  ( -7.895350322657909814, -8.000000000000000000, -398.4775300148394308 ) ) ;
#8963=EDGE_CURVE ( 'NONE', #5389, #1717, #6069, .T. ) ;
#8971=FILL_AREA_STYLE_COLOUR ( '', #5048 ) ;
#8972=DIRECTION ( 'NONE',  ( -0.1071946444232961260, 0.000000000000000000, 0.9942380540931650135 ) ) ;
#8995=CARTESIAN_POINT ( 'NONE',  ( -3.339933055294987074, -9.500000000000001776, -397.0720243238112630 ) ) ;
#8998=CARTESIAN_POINT ( 'NONE',  ( -2.000000000003786749, -8.000000000000000000, -409.4999999999758415 ) ) ;
#9004=CARTESIAN_POINT ( 'NONE',  ( -43.46674421124934184, -8.000000000000000000, -402.7790142173016648 ) ) ;
#9009=AXIS2_PLACEMENT_3D ( 'NONE', #1077, #5363, #6789 ) ;
#9021=( LENGTH_UNIT ( ) NAMED_UNIT ( * ) SI_UNIT ( .MILLI., .METRE. ) );
#9027=ORIENTED_EDGE ( 'NONE', *, *, #5385, .F. ) ;
#9072=CARTESIAN_POINT ( 'NONE',  ( -2.000000000003786749, -7.500000000000000888, -409.4999999999758415 ) ) ;
#9074=( NAMED_UNIT ( * ) PLANE_ANGLE_UNIT ( ) SI_UNIT ( $, .RADIAN. ) );
#9082=ORIENTED_EDGE ( 'NONE', *, *, #7851, .F. ) ;
#9093=EDGE_CURVE ( 'NONE', #6915, #10437, #4367, .T. ) ;
#9094=DIRECTION ( 'NONE',  ( 0.000000000000000000, 1.000000000000000000, 0.000000000000000000 ) ) ;
#9099=ADVANCED_FACE ( 'NONE', ( #10314 ), #1336, .F. ) ;
#9110=ORIENTED_EDGE ( 'NONE', *, *, #2451, .F. ) ;
#9132=DIRECTION ( 'NONE',  ( -0.9942380540931649024, 0.000000000000000000, -0.1071946444232959872 ) ) ;
#9157=FACE_OUTER_BOUND ( 'NONE', #8040, .T. ) ;
#9170=ORIENTED_EDGE ( 'NONE', *, *, #7309, .F. ) ;
#9172=EDGE_CURVE ( 'NONE', #6903, #4635, #3677, .T. ) ;
#9195=VECTOR ( 'NONE', #9132, 1000.000000000000114 ) ;
#9201=DIRECTION ( 'NONE',  ( 0.000000000000000000, -1.000000000000000000, 0.000000000000000000 ) ) ;
#9207=DIRECTION ( 'NONE',  ( 0.000000000000000000, 1.000000000000000000, 0.000000000000000000 ) ) ;
#9208=EDGE_LOOP ( 'NONE', ( #5456, #3420, #4032, #7400 ) ) ;
#9218=EDGE_LOOP ( 'NONE', ( #8889, #8681, #7226, #2724, #3073, #9110 ) ) ;
#9222=AXIS2_PLACEMENT_3D ( 'NONE', #3508, #9565, #4679 ) ;
#9232=ORIENTED_EDGE ( 'NONE', *, *, #7054, .T. ) ;
#9238=ADVANCED_FACE ( 'NONE', ( #2470 ), #5520, .T. ) ;
#9240=( NAMED_UNIT ( * ) PLANE_ANGLE_UNIT ( ) SI_UNIT ( $, .RADIAN. ) );
#9241=DIRECTION ( 'NONE',  ( 0.000000000000000000, 1.000000000000000000, 0.000000000000000000 ) ) ;
#9253=CARTESIAN_POINT ( 'NONE',  ( -13.36185104352900055, -9.000000000000001776, -400.1641368440791098 ) ) ;
#9262=CARTESIAN_POINT ( 'NONE',  ( -26.31853765676889267, -9.000000000000001776, -432.7407288192795249 ) ) ;
#9286=DIRECTION ( 'NONE',  ( 0.9942380540931650135, 0.000000000000000000, 0.1071946444232960011 ) ) ;
#9300=CARTESIAN_POINT ( 'NONE',  ( -47.11589368967775471, -7.500000000000000888, -410.8439258096980780 ) ) ;
#9302=ADVANCED_FACE ( 'NONE', ( #1662, #8803, #4785 ), #4731, .T. ) ;
#9303=CARTESIAN_POINT ( 'NONE',  ( -27.98005464532998232, -9.500000000000001776, -417.3300389808354680 ) ) ;
#9306=DIRECTION ( 'NONE',  ( -0.4716280258120416069, 0.000000000000000000, 0.8817975988108813779 ) ) ;
#9307=DIRECTION ( 'NONE',  ( 0.9942380540931625710, 0.000000000000000000, 0.1071946444233177614 ) ) ;
#9308=CARTESIAN_POINT ( 'NONE',  ( -18.02719435607597021, -9.500000000000001776, -431.8467903975401896 ) ) ;
#9310=CARTESIAN_POINT ( 'NONE',  ( -27.92645732311634532, -9.000000000000001776, -417.8271580078818488 ) ) ;
#9314=CARTESIAN_POINT ( 'NONE',  ( -1.624818744522249503, -9.500000000000001776, -412.9798331893018712 ) ) ;
#9326=AXIS2_PLACEMENT_3D ( 'NONE', #51, #5786, #7251 ) ;
#9340=AXIS2_PLACEMENT_3D ( 'NONE', #8254, #893, #259 ) ;
#9355=LINE ( 'NONE', #1990, #5701 ) ;
#9376=VERTEX_POINT ( 'NONE', #3154 ) ;
#9388=CARTESIAN_POINT ( 'NONE',  ( -43.46674421124934184, -7.500000000000000888, -402.7790142173016648 ) ) ;
#9399=ORIENTED_EDGE ( 'NONE', *, *, #543, .T. ) ;
#9436=CARTESIAN_POINT ( 'NONE',  ( -18.02719435607597021, -9.633703999999999823, -431.8467903975401896 ) ) ;
#9439=FACE_OUTER_BOUND ( 'NONE', #7009, .T. ) ;
#9471=ORIENTED_EDGE ( 'NONE', *, *, #5504, .T. ) ;
#9485=DIRECTION ( 'NONE',  ( 0.000000000000000000, 1.000000000000000000, 0.000000000000000000 ) ) ;
#9486=DIRECTION ( 'NONE',  ( -0.1071946444232964035, 0.000000000000000000, 0.9942380540931649024 ) ) ;
#9491=EDGE_CURVE ( 'NONE', #3077, #5506, #2489, .T. ) ;
#9510=AXIS2_PLACEMENT_3D ( 'NONE', #1624, #809, #4092 ) ;
#9515=ORIENTED_EDGE ( 'NONE', *, *, #3125, .F. ) ;
#9533=MECHANICAL_DESIGN_GEOMETRIC_PRESENTATION_REPRESENTATION('',(#784),#5931);
#9557=FACE_OUTER_BOUND ( 'NONE', #8775, .T. ) ;
#9561=DIRECTION ( 'NONE',  ( 0.9942380540931649024, 0.000000000000000000, 0.1071946444232959872 ) ) ;
#9565=DIRECTION ( 'NONE',  ( 0.8126105599114364919, 0.000000000000000000, -0.5828070674935419415 ) ) ;
#9589=ORIENTED_EDGE ( 'NONE', *, *, #2683, .T. ) ;
#9599=CARTESIAN_POINT ( 'NONE',  ( -2.000000000003786749, -9.000000000000001776, -409.4999999999758415 ) ) ;
#9605=EDGE_CURVE ( 'NONE', #3194, #1259, #10553, .T. ) ;
#9614=ORIENTED_EDGE ( 'NONE', *, *, #7911, .T. ) ;
#9624=CYLINDRICAL_SURFACE ( 'NONE', #6610, 3.500000000000020428 ) ;
#9625=EDGE_CURVE ( 'NONE', #10492, #7240, #10037, .T. ) ;
#9635=CARTESIAN_POINT ( 'NONE',  ( -2.000000000003786749, -9.500000000000001776, -409.4999999999758415 ) ) ;
#9637=LINE ( 'NONE', #8995, #511 ) ;
#9639=VERTEX_POINT ( 'NONE', #10182 ) ;
#9646=FACE_OUTER_BOUND ( 'NONE', #10180, .T. ) ;
#9665=( LENGTH_UNIT ( ) NAMED_UNIT ( * ) SI_UNIT ( .MILLI., .METRE. ) );
#9679=CARTESIAN_POINT ( 'NONE',  ( -18.02719435607597021, -9.000000000000001776, -431.8467903975401896 ) ) ;
#9693=DIRECTION ( 'NONE',  ( 0.000000000000000000, -1.000000000000000000, 0.000000000000000000 ) ) ;
#9704=CARTESIAN_POINT ( 'NONE',  ( -46.74071243419621169, -9.500000000000001776, -414.3237589990241077 ) ) ;
#9706=DIRECTION ( 'NONE',  ( -0.1071946444232958900, 0.000000000000000000, 0.9942380540931649024 ) ) ;
#9716=CARTESIAN_POINT ( 'NONE',  ( -0.6600669447125837586, -8.000000000000000000, -421.9279756761403632 ) ) ;
#9721=LINE ( 'NONE', #2466, #4850 ) ;
#9724=FILL_AREA_STYLE ('',( #8971 ) ) ;
#9735=DIRECTION ( 'NONE',  ( 0.4716280258120408853, 0.000000000000000000, -0.8817975988108818219 ) ) ;
#9743=ORIENTED_EDGE ( 'NONE', *, *, #6736, .T. ) ;
#9749=ORIENTED_EDGE ( 'NONE', *, *, #4906, .T. ) ;
#9753=ORIENTED_EDGE ( 'NONE', *, *, #2451, .T. ) ;
#9757=CARTESIAN_POINT ( 'NONE',  ( -2.000000000003786749, -9.000000000000001776, -409.4999999999758415 ) ) ;
#9772=( NAMED_UNIT ( * ) SI_UNIT ( $, .STERADIAN. ) SOLID_ANGLE_UNIT ( ) );
#9777=CARTESIAN_POINT ( 'NONE',  ( -18.02719435607597021, -8.000000000000000000, -431.8467903975401896 ) ) ;
#9790=DIRECTION ( 'NONE',  ( -0.1173809667161559989, 0.000000000000000000, 0.9930869592602555862 ) ) ;
#9804=ORIENTED_EDGE ( 'NONE', *, *, #5800, .T. ) ;
#9814=ORIENTED_EDGE ( 'NONE', *, *, #8963, .T. ) ;
#9858=ORIENTED_EDGE ( 'NONE', *, *, #554, .F. ) ;
#9860=AXIS2_PLACEMENT_3D ( 'NONE', #9679, #4744, #9790 ) ;
#9875=EDGE_LOOP ( 'NONE', ( #9753, #3732, #7441, #5444, #9743, #1770, #3327, #622 ) ) ;
#9879=DIRECTION ( 'NONE',  ( 0.1071946444232954182, 0.000000000000000000, -0.9942380540931651245 ) ) ;
#9900=ADVANCED_FACE ( 'NONE', ( #9157 ), #3861, .T. ) ;
#9927=LINE ( 'NONE', #204, #4700 ) ;
#9928=DIRECTION ( 'NONE',  ( 1.477360691113388328E-12, 1.000000000000000000, 1.592829336162332234E-13 ) ) ;
#9937=ORIENTED_EDGE ( 'NONE', *, *, #7909, .F. ) ;
#9955=AXIS2_PLACEMENT_3D ( 'NONE', #8049, #3219, #1555 ) ;
#9959=CARTESIAN_POINT ( 'NONE',  ( -19.68871134463705985, -8.000000000000000000, -416.4361005590961327 ) ) ;
#9965=DIRECTION ( 'NONE',  ( 0.000000000000000000, 1.000000000000000000, 0.000000000000000000 ) ) ;
#10009=DIRECTION ( 'NONE',  ( 0.000000000000000000, -1.000000000000000000, 0.000000000000000000 ) ) ;
#10010=CARTESIAN_POINT ( 'NONE',  ( -18.02719435607597021, -8.000000000000000000, -431.8467903975401896 ) ) ;
#10015=EDGE_LOOP ( 'NONE', ( #7089, #7334, #9515, #854 ) ) ;
#10018=VERTEX_POINT ( 'NONE', #6900 ) ;
#10033=CYLINDRICAL_SURFACE ( 'NONE', #8130, 12.49999999999998757 ) ;
#10037=CIRCLE ( 'NONE', #5058, 15.50000000000001421 ) ;
#10050=EDGE_CURVE ( 'NONE', #6593, #24, #1975, .T. ) ;
#10102=DIRECTION ( 'NONE',  ( -0.8817975988108817109, 2.326394606397485120E-15, -0.4716280258120411073 ) ) ;
#10105=LINE ( 'NONE', #2747, #2309 ) ;
#10109=DIRECTION ( 'NONE',  ( 0.000000000000000000, -1.000000000000000000, 0.000000000000000000 ) ) ;
#10131=VERTEX_POINT ( 'NONE', #8959 ) ;
#10135=CARTESIAN_POINT ( 'NONE',  ( -43.46674421124934184, -9.500000000000001776, -402.7790142173016648 ) ) ;
#10156=ADVANCED_FACE ( 'NONE', ( #5994 ), #8307, .T. ) ;
#10170=CARTESIAN_POINT ( 'NONE',  ( -7.659536309752155603, -9.500000000000001776, -398.9184288142485570 ) ) ;
#10180=EDGE_LOOP ( 'NONE', ( #930, #2587, #6742, #5185, #9937, #10433 ) ) ;
#10182=CARTESIAN_POINT ( 'NONE',  ( -37.57635160138833896, -9.500000000000001776, -403.2777420460153053 ) ) ;
#10187=ORIENTED_EDGE ( 'NONE', *, *, #7054, .F. ) ;
#10188=CYLINDRICAL_SURFACE ( 'NONE', #1782, 15.00000000000001776 ) ;
#10200=ORIENTED_EDGE ( 'NONE', *, *, #8619, .T. ) ;
#10216=CARTESIAN_POINT ( 'NONE',  ( -46.36553117871467578, -7.500000000000000888, -417.8035921883502510 ) ) ;
#10218=EDGE_CURVE ( 'NONE', #10253, #7180, #2121, .T. ) ;
#10227=EDGE_CURVE ( 'NONE', #4863, #3194, #9927, .T. ) ;
#10232=ORIENTED_EDGE ( 'NONE', *, *, #10530, .F. ) ;
#10236=DIRECTION ( 'NONE',  ( 0.09270529807100655328, 0.000000000000000000, -0.9956935912767369556 ) ) ;
#10253=VERTEX_POINT ( 'NONE', #5831 ) ;
#10258=TOROIDAL_SURFACE ( 'NONE', #6299, 15.50000000000000000, 0.5000000000000000000 ) ;
#10271=DIRECTION ( 'NONE',  ( 0.000000000000000000, -1.000000000000000000, 0.000000000000000000 ) ) ;
#10272=ADVANCED_FACE ( 'NONE', ( #6761 ), #10033, .T. ) ;
#10273=DIRECTION ( 'NONE',  ( 0.000000000000000000, -1.000000000000000000, 0.000000000000000000 ) ) ;
#10314=FACE_OUTER_BOUND ( 'NONE', #8786, .T. ) ;
#10318=ORIENTED_EDGE ( 'NONE', *, *, #3468, .F. ) ;
#10331=PRODUCT ( 'Secondary Linkage Connector', 'Secondary Linkage Connector', '', ( #2374 ) ) ;
#10334=CIRCLE ( 'NONE', #3993, 12.50000000000002309 ) ;
#10338=EDGE_CURVE ( 'NONE', #10018, #6553, #8811, .T. ) ;
#10347=ORIENTED_EDGE ( 'NONE', *, *, #2013, .T. ) ;
#10354=ORIENTED_EDGE ( 'NONE', *, *, #7939, .F. ) ;
#10365=AXIS2_PLACEMENT_3D ( 'NONE', #6889, #7736, #7948 ) ;
#10366=CARTESIAN_POINT ( 'NONE',  ( -48.08064548948741646, -9.000000000000001776, -401.8957833228595860 ) ) ;
#10385=DIRECTION ( 'NONE',  ( 0.9942380540931649024, 0.000000000000000000, 0.1071946444232959872 ) ) ;
#10408=VERTEX_POINT ( 'NONE', #9388 ) ;
#10414=SURFACE_STYLE_FILL_AREA ( #9724 ) ;
#10415=CARTESIAN_POINT ( 'NONE',  ( -2.000000000003786749, -9.500000000000001776, -409.4999999999758415 ) ) ;
#10422=ADVANCED_FACE ( 'NONE', ( #517 ), #10188, .F. ) ;
#10433=ORIENTED_EDGE ( 'NONE', *, *, #6585, .F. ) ;
#10437=VERTEX_POINT ( 'NONE', #4439 ) ;
#10464=DIRECTION ( 'NONE',  ( -6.627266684903556796E-12, 1.000000000000000000, 1.877906674862047561E-12 ) ) ;
#10479=EDGE_CURVE ( 'NONE', #2787, #1717, #69, .T. ) ;
#10492=VERTEX_POINT ( 'NONE', #1260 ) ;
#10518=PLANE ( 'NONE',  #7042 ) ;
#10527=CARTESIAN_POINT ( 'NONE',  ( -9.285088343770869557, -9.000000000000001776, -419.6576319987959778 ) ) ;
#10530=EDGE_CURVE ( 'NONE', #1489, #6903, #3051, .T. ) ;
#10540=CIRCLE ( 'NONE', #3675, 0.5000000000000004441 ) ;
#10546=AXIS2_PLACEMENT_3D ( 'NONE', #3713, #4510, #8538 ) ;
#10553=CIRCLE ( 'NONE', #4378, 3.500000000000020428 ) ;
#10557=ORIENTED_EDGE ( 'NONE', *, *, #181, .F. ) ;
#10582=DIRECTION ( 'NONE',  ( 0.000000000000000000, -1.000000000000000000, 0.000000000000000000 ) ) ;
#10590=FACE_OUTER_BOUND ( 'NONE', #8166, .T. ) ;
#10591=FACE_OUTER_BOUND ( 'NONE', #2486, .T. ) ;
#10600=CIRCLE ( 'NONE', #1858, 0.5000000000000004441 ) ;
#10607=ORIENTED_EDGE ( 'NONE', *, *, #5217, .F. ) ;
ENDSEC;
END-ISO-10303-21;
